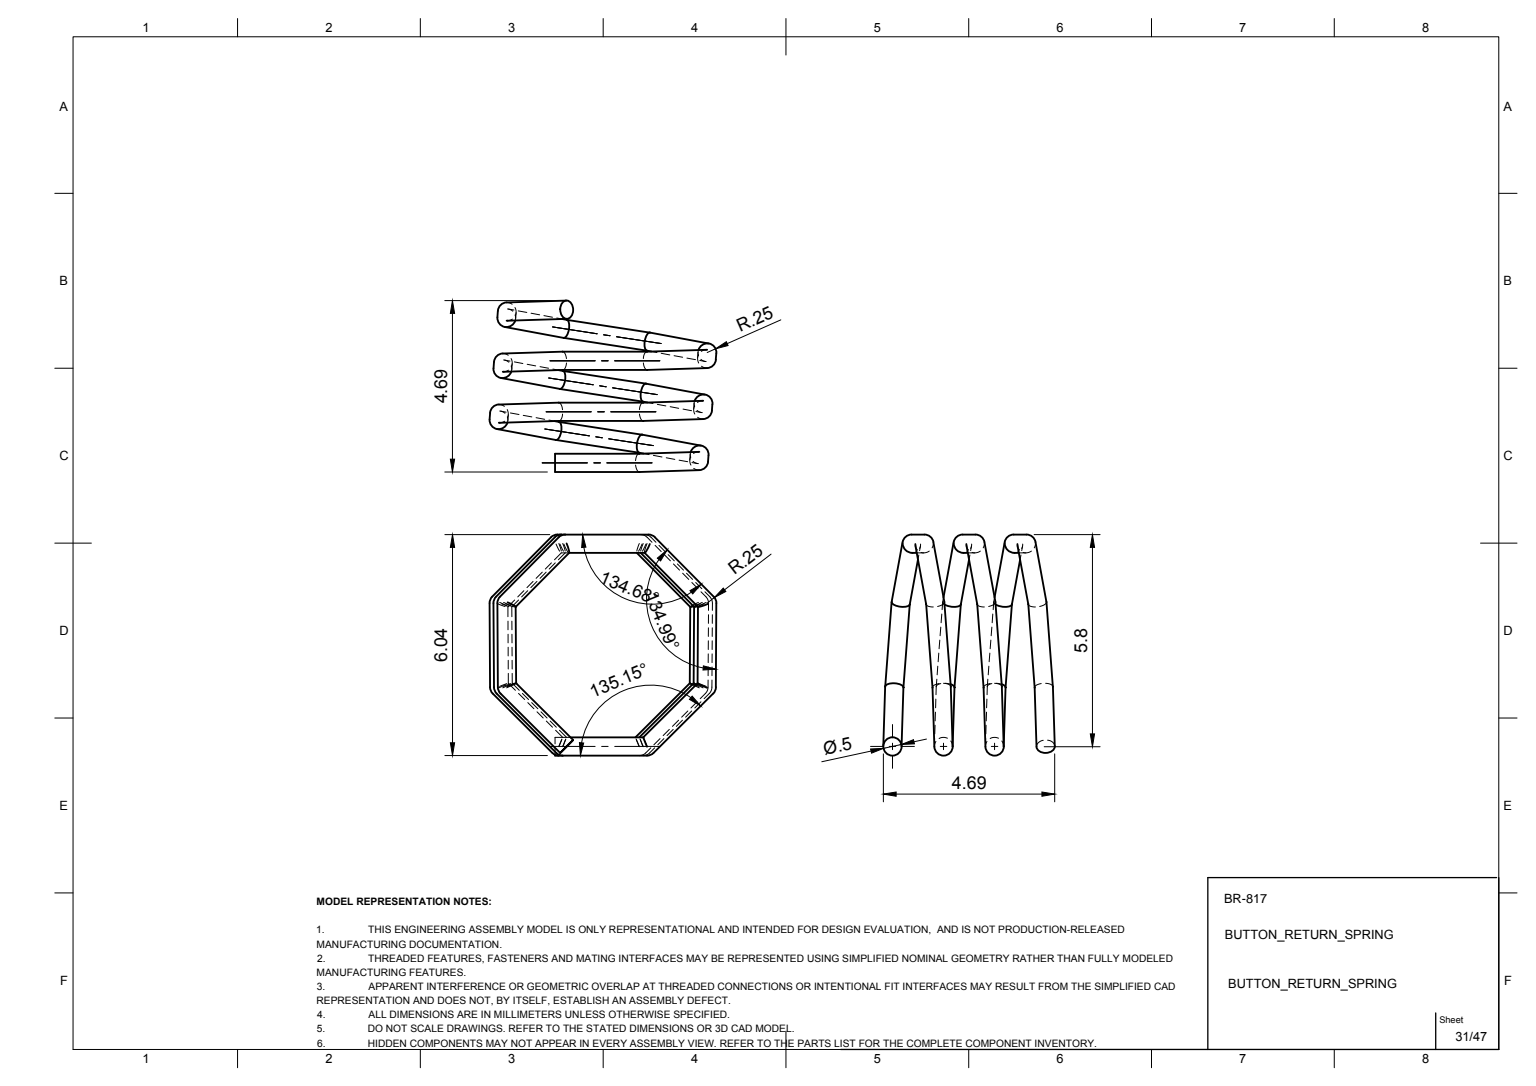
ISO-10303-21;
HEADER;
FILE_DESCRIPTION((''),'2;1');
FILE_NAME('BUTTON_RETURN_SPRING.step','2026-10-01T22:07:29-07:00',(''),(''),'','','');
FILE_SCHEMA (('AUTOMOTIVE_DESIGN { 1 0 10303 214 3 1 1 }'));
ENDSEC;
DATA;
#10=MECHANICAL_DESIGN_GEOMETRIC_PRESENTATION_REPRESENTATION('',(#563),#15484);
#88=ELLIPSE('',#9445,0.0270464082562617,0.025) ;
#89=ELLIPSE('',#9446,0.0270464082562617,0.025) ;
#90=ELLIPSE('',#9447,0.0270464082562617,0.025) ;
#91=ELLIPSE('',#9450,0.0270464082562613,0.025) ;
#92=ELLIPSE('',#9451,0.0270464082562613,0.025) ;
#93=ELLIPSE('',#9453,0.0270464082562612,0.025) ;
#94=ELLIPSE('',#9455,0.0270464082562616,0.025) ;
#95=ELLIPSE('',#9457,0.0270464082562615,0.025) ;
#96=ELLIPSE('',#9459,0.0270464082562615,0.025) ;
#97=ELLIPSE('',#9460,0.0270464082562615,0.025) ;
#98=ELLIPSE('',#9462,0.0270464082562615,0.025) ;
#99=ELLIPSE('',#9463,0.0270464082562615,0.025) ;
#100=ELLIPSE('',#9464,0.0270464082562615,0.025) ;
#101=ELLIPSE('',#9466,0.0270464082562616,0.025) ;
#102=ELLIPSE('',#9467,0.0270464082562616,0.025) ;
#103=ELLIPSE('',#9469,0.0270464082562617,0.025) ;
#104=ELLIPSE('',#9470,0.0270464082562617,0.025) ;
#105=ELLIPSE('',#9471,0.0270464082562617,0.025) ;
#106=ELLIPSE('',#9473,0.0270464082562615,0.025) ;
#107=ELLIPSE('',#9474,0.0270464082562615,0.025) ;
#108=ELLIPSE('',#9476,0.0270464082562614,0.025) ;
#109=ELLIPSE('',#9478,0.0270464082562616,0.025) ;
#110=ELLIPSE('',#9480,0.0270464082562617,0.025) ;
#111=ELLIPSE('',#9482,0.0270464082562615,0.025) ;
#112=ELLIPSE('',#9483,0.0270464082562615,0.025) ;
#113=ELLIPSE('',#9485,0.0270464082562615,0.025) ;
#114=ELLIPSE('',#9486,0.0270464082562615,0.025) ;
#115=ELLIPSE('',#9487,0.0270464082562615,0.025) ;
#116=ELLIPSE('',#9489,0.0270464082562617,0.025) ;
#117=ELLIPSE('',#9490,0.0270464082562617,0.025) ;
#118=ELLIPSE('',#9492,0.0270464082562616,0.025) ;
#119=ELLIPSE('',#9493,0.0270464082562616,0.025) ;
#120=ELLIPSE('',#9494,0.0270464082562616,0.025) ;
#121=ELLIPSE('',#9496,0.0270464082562616,0.025) ;
#122=ELLIPSE('',#9497,0.0270464082562616,0.025) ;
#123=ELLIPSE('',#9499,0.0270464082562614,0.025) ;
#124=ELLIPSE('',#9501,0.0270464082562616,0.025) ;
#125=ELLIPSE('',#9503,0.0270464082562616,0.025) ;
#126=ELLIPSE('',#9505,0.0270464082562616,0.025) ;
#127=ELLIPSE('',#9506,0.0270464082562616,0.025) ;
#128=ELLIPSE('',#9508,0.0270464082562615,0.025) ;
#129=ELLIPSE('',#9509,0.0270464082562615,0.025) ;
#130=ELLIPSE('',#9510,0.0270464082562615,0.025) ;
#237=SPHERICAL_SURFACE('',#9350,0.025) ;
#238=SPHERICAL_SURFACE('',#9353,0.025) ;
#239=SPHERICAL_SURFACE('',#9357,0.025) ;
#240=SPHERICAL_SURFACE('',#9362,0.025) ;
#241=SPHERICAL_SURFACE('',#9367,0.025) ;
#242=SPHERICAL_SURFACE('',#9372,0.025) ;
#243=SPHERICAL_SURFACE('',#9376,0.025) ;
#244=SPHERICAL_SURFACE('',#9379,0.025) ;
#245=SPHERICAL_SURFACE('',#9382,0.025) ;
#246=SPHERICAL_SURFACE('',#9385,0.025) ;
#247=SPHERICAL_SURFACE('',#9389,0.025) ;
#248=SPHERICAL_SURFACE('',#9394,0.025) ;
#249=SPHERICAL_SURFACE('',#9399,0.025) ;
#250=SPHERICAL_SURFACE('',#9404,0.025) ;
#251=SPHERICAL_SURFACE('',#9408,0.025) ;
#252=SPHERICAL_SURFACE('',#9411,0.025) ;
#253=SPHERICAL_SURFACE('',#9414,0.025) ;
#254=SPHERICAL_SURFACE('',#9417,0.025) ;
#255=SPHERICAL_SURFACE('',#9421,0.025) ;
#256=SPHERICAL_SURFACE('',#9426,0.025) ;
#257=SPHERICAL_SURFACE('',#9431,0.025) ;
#258=SPHERICAL_SURFACE('',#9436,0.025) ;
#259=SPHERICAL_SURFACE('',#9440,0.025) ;
#493=SHAPE_REPRESENTATION_RELATIONSHIP('SRR','None',#15643,#528) ;
#528=ADVANCED_BREP_SHAPE_REPRESENTATION('',(#604),#15467) ;
#563=STYLED_ITEM('',(#15832),#604) ;
#604=MANIFOLD_SOLID_BREP('BUTTON_RETURN_SPRING',#8274) ;
#732=CYLINDRICAL_SURFACE('',#9443,0.025) ;
#733=CYLINDRICAL_SURFACE('',#9449,0.025) ;
#734=CYLINDRICAL_SURFACE('',#9452,0.025) ;
#735=CYLINDRICAL_SURFACE('',#9454,0.025) ;
#736=CYLINDRICAL_SURFACE('',#9456,0.025) ;
#737=CYLINDRICAL_SURFACE('',#9458,0.025) ;
#738=CYLINDRICAL_SURFACE('',#9461,0.025) ;
#739=CYLINDRICAL_SURFACE('',#9465,0.025) ;
#740=CYLINDRICAL_SURFACE('',#9468,0.025) ;
#741=CYLINDRICAL_SURFACE('',#9472,0.025) ;
#742=CYLINDRICAL_SURFACE('',#9475,0.025) ;
#743=CYLINDRICAL_SURFACE('',#9477,0.025) ;
#744=CYLINDRICAL_SURFACE('',#9479,0.025) ;
#745=CYLINDRICAL_SURFACE('',#9481,0.025) ;
#746=CYLINDRICAL_SURFACE('',#9484,0.025) ;
#747=CYLINDRICAL_SURFACE('',#9488,0.025) ;
#748=CYLINDRICAL_SURFACE('',#9491,0.025) ;
#749=CYLINDRICAL_SURFACE('',#9495,0.025) ;
#750=CYLINDRICAL_SURFACE('',#9498,0.025) ;
#751=CYLINDRICAL_SURFACE('',#9500,0.025) ;
#752=CYLINDRICAL_SURFACE('',#9502,0.025) ;
#753=CYLINDRICAL_SURFACE('',#9504,0.025) ;
#754=CYLINDRICAL_SURFACE('',#9507,0.025) ;
#755=CYLINDRICAL_SURFACE('',#9511,0.025) ;
#1147=CIRCLE('',#9351,0.025) ;
#1148=CIRCLE('',#9352,0.025) ;
#1149=CIRCLE('',#9354,0.025) ;
#1150=CIRCLE('',#9355,0.025) ;
#1151=CIRCLE('',#9356,0.025) ;
#1152=CIRCLE('',#9358,0.025) ;
#1153=CIRCLE('',#9359,0.025) ;
#1154=CIRCLE('',#9360,0.025) ;
#1155=CIRCLE('',#9361,0.025) ;
#1156=CIRCLE('',#9363,0.025) ;
#1157=CIRCLE('',#9364,0.025) ;
#1158=CIRCLE('',#9365,0.025) ;
#1159=CIRCLE('',#9366,0.025) ;
#1160=CIRCLE('',#9368,0.025) ;
#1161=CIRCLE('',#9369,0.025) ;
#1162=CIRCLE('',#9370,0.025) ;
#1163=CIRCLE('',#9371,0.025) ;
#1164=CIRCLE('',#9373,0.025) ;
#1165=CIRCLE('',#9374,0.025) ;
#1166=CIRCLE('',#9375,0.025) ;
#1167=CIRCLE('',#9377,0.025) ;
#1168=CIRCLE('',#9378,0.025) ;
#1169=CIRCLE('',#9380,0.025) ;
#1170=CIRCLE('',#9381,0.025) ;
#1171=CIRCLE('',#9383,0.025) ;
#1172=CIRCLE('',#9384,0.025) ;
#1173=CIRCLE('',#9386,0.025) ;
#1174=CIRCLE('',#9387,0.025) ;
#1175=CIRCLE('',#9388,0.025) ;
#1176=CIRCLE('',#9390,0.025) ;
#1177=CIRCLE('',#9391,0.025) ;
#1178=CIRCLE('',#9392,0.025) ;
#1179=CIRCLE('',#9393,0.025) ;
#1180=CIRCLE('',#9395,0.025) ;
#1181=CIRCLE('',#9396,0.025) ;
#1182=CIRCLE('',#9397,0.025) ;
#1183=CIRCLE('',#9398,0.025) ;
#1184=CIRCLE('',#9400,0.025) ;
#1185=CIRCLE('',#9401,0.025) ;
#1186=CIRCLE('',#9402,0.025) ;
#1187=CIRCLE('',#9403,0.025) ;
#1188=CIRCLE('',#9405,0.025) ;
#1189=CIRCLE('',#9406,0.025) ;
#1190=CIRCLE('',#9407,0.025) ;
#1191=CIRCLE('',#9409,0.025) ;
#1192=CIRCLE('',#9410,0.025) ;
#1193=CIRCLE('',#9412,0.025) ;
#1194=CIRCLE('',#9413,0.025) ;
#1195=CIRCLE('',#9415,0.025) ;
#1196=CIRCLE('',#9416,0.025) ;
#1197=CIRCLE('',#9418,0.025) ;
#1198=CIRCLE('',#9419,0.025) ;
#1199=CIRCLE('',#9420,0.025) ;
#1200=CIRCLE('',#9422,0.025) ;
#1201=CIRCLE('',#9423,0.025) ;
#1202=CIRCLE('',#9424,0.025) ;
#1203=CIRCLE('',#9425,0.025) ;
#1204=CIRCLE('',#9427,0.025) ;
#1205=CIRCLE('',#9428,0.025) ;
#1206=CIRCLE('',#9429,0.025) ;
#1207=CIRCLE('',#9430,0.025) ;
#1208=CIRCLE('',#9432,0.025) ;
#1209=CIRCLE('',#9433,0.025) ;
#1210=CIRCLE('',#9434,0.025) ;
#1211=CIRCLE('',#9435,0.025) ;
#1212=CIRCLE('',#9437,0.025) ;
#1213=CIRCLE('',#9438,0.025) ;
#1214=CIRCLE('',#9439,0.025) ;
#1215=CIRCLE('',#9441,0.025) ;
#1216=CIRCLE('',#9442,0.025) ;
#1217=CIRCLE('',#9444,0.025) ;
#1218=CIRCLE('',#9512,0.025) ;
#1655=FACE_OUTER_BOUND('',#2220,.T.) ;
#1656=FACE_OUTER_BOUND('',#2221,.T.) ;
#1657=FACE_OUTER_BOUND('',#2222,.T.) ;
#1658=FACE_OUTER_BOUND('',#2223,.T.) ;
#1659=FACE_OUTER_BOUND('',#2224,.T.) ;
#1660=FACE_OUTER_BOUND('',#2225,.T.) ;
#1661=FACE_OUTER_BOUND('',#2226,.T.) ;
#1662=FACE_OUTER_BOUND('',#2227,.T.) ;
#1663=FACE_OUTER_BOUND('',#2228,.T.) ;
#1664=FACE_OUTER_BOUND('',#2229,.T.) ;
#1665=FACE_OUTER_BOUND('',#2230,.T.) ;
#1666=FACE_OUTER_BOUND('',#2231,.T.) ;
#1667=FACE_OUTER_BOUND('',#2232,.T.) ;
#1668=FACE_OUTER_BOUND('',#2233,.T.) ;
#1669=FACE_OUTER_BOUND('',#2234,.T.) ;
#1670=FACE_OUTER_BOUND('',#2235,.T.) ;
#1671=FACE_OUTER_BOUND('',#2236,.T.) ;
#1672=FACE_OUTER_BOUND('',#2237,.T.) ;
#1673=FACE_OUTER_BOUND('',#2238,.T.) ;
#1674=FACE_OUTER_BOUND('',#2239,.T.) ;
#1675=FACE_OUTER_BOUND('',#2240,.T.) ;
#1676=FACE_OUTER_BOUND('',#2241,.T.) ;
#1677=FACE_OUTER_BOUND('',#2242,.T.) ;
#1678=FACE_OUTER_BOUND('',#2243,.T.) ;
#1679=FACE_OUTER_BOUND('',#2244,.T.) ;
#1680=FACE_OUTER_BOUND('',#2245,.T.) ;
#1681=FACE_OUTER_BOUND('',#2246,.T.) ;
#1682=FACE_OUTER_BOUND('',#2247,.T.) ;
#1683=FACE_OUTER_BOUND('',#2248,.T.) ;
#1684=FACE_OUTER_BOUND('',#2249,.T.) ;
#1685=FACE_OUTER_BOUND('',#2250,.T.) ;
#1686=FACE_OUTER_BOUND('',#2251,.T.) ;
#1687=FACE_OUTER_BOUND('',#2252,.T.) ;
#1688=FACE_OUTER_BOUND('',#2253,.T.) ;
#1689=FACE_OUTER_BOUND('',#2254,.T.) ;
#1690=FACE_OUTER_BOUND('',#2255,.T.) ;
#1691=FACE_OUTER_BOUND('',#2256,.T.) ;
#1692=FACE_OUTER_BOUND('',#2257,.T.) ;
#1693=FACE_OUTER_BOUND('',#2258,.T.) ;
#1694=FACE_OUTER_BOUND('',#2259,.T.) ;
#1695=FACE_OUTER_BOUND('',#2260,.T.) ;
#1696=FACE_OUTER_BOUND('',#2261,.T.) ;
#1697=FACE_OUTER_BOUND('',#2262,.T.) ;
#1698=FACE_OUTER_BOUND('',#2263,.T.) ;
#1699=FACE_OUTER_BOUND('',#2264,.T.) ;
#1700=FACE_OUTER_BOUND('',#2265,.T.) ;
#1701=FACE_OUTER_BOUND('',#2266,.T.) ;
#1702=FACE_OUTER_BOUND('',#2267,.T.) ;
#1703=FACE_OUTER_BOUND('',#2268,.T.) ;
#2220=EDGE_LOOP('',(#6565,#6566)) ;
#2221=EDGE_LOOP('',(#6567,#6568,#6569)) ;
#2222=EDGE_LOOP('',(#6570,#6571,#6572,#6573)) ;
#2223=EDGE_LOOP('',(#6574,#6575,#6576,#6577)) ;
#2224=EDGE_LOOP('',(#6578,#6579,#6580,#6581)) ;
#2225=EDGE_LOOP('',(#6582,#6583,#6584)) ;
#2226=EDGE_LOOP('',(#6585,#6586)) ;
#2227=EDGE_LOOP('',(#6587,#6588)) ;
#2228=EDGE_LOOP('',(#6589,#6590)) ;
#2229=EDGE_LOOP('',(#6591,#6592,#6593)) ;
#2230=EDGE_LOOP('',(#6594,#6595,#6596,#6597)) ;
#2231=EDGE_LOOP('',(#6598,#6599,#6600,#6601)) ;
#2232=EDGE_LOOP('',(#6602,#6603,#6604,#6605)) ;
#2233=EDGE_LOOP('',(#6606,#6607,#6608)) ;
#2234=EDGE_LOOP('',(#6609,#6610)) ;
#2235=EDGE_LOOP('',(#6611,#6612)) ;
#2236=EDGE_LOOP('',(#6613,#6614)) ;
#2237=EDGE_LOOP('',(#6615,#6616,#6617)) ;
#2238=EDGE_LOOP('',(#6618,#6619,#6620,#6621)) ;
#2239=EDGE_LOOP('',(#6622,#6623,#6624,#6625)) ;
#2240=EDGE_LOOP('',(#6626,#6627,#6628,#6629)) ;
#2241=EDGE_LOOP('',(#6630,#6631,#6632)) ;
#2242=EDGE_LOOP('',(#6633,#6634)) ;
#2243=EDGE_LOOP('',(#6635,#6636,#6637,#6638,#6639,#6640,#6641)) ;
#2244=EDGE_LOOP('',(#6642)) ;
#2245=EDGE_LOOP('',(#6643,#6644,#6645,#6646,#6647,#6648,#6649,#6650,#6651)) ;
#2246=EDGE_LOOP('',(#6652,#6653,#6654,#6655,#6656,#6657,#6658,#6659,#6660)) ;
#2247=EDGE_LOOP('',(#6661,#6662,#6663,#6664,#6665,#6666,#6667,#6668)) ;
#2248=EDGE_LOOP('',(#6669,#6670,#6671,#6672,#6673,#6674,#6675,#6676)) ;
#2249=EDGE_LOOP('',(#6677,#6678,#6679,#6680,#6681,#6682,#6683,#6684,#6685)) ;
#2250=EDGE_LOOP('',(#6686,#6687,#6688,#6689,#6690,#6691,#6692,#6693,#6694)) ;
#2251=EDGE_LOOP('',(#6695,#6696,#6697,#6698,#6699,#6700,#6701,#6702,#6703)) ;
#2252=EDGE_LOOP('',(#6704,#6705,#6706,#6707,#6708,#6709,#6710,#6711,#6712)) ;
#2253=EDGE_LOOP('',(#6713,#6714,#6715,#6716,#6717,#6718,#6719,#6720,#6721)) ;
#2254=EDGE_LOOP('',(#6722,#6723,#6724,#6725,#6726,#6727,#6728,#6729,#6730)) ;
#2255=EDGE_LOOP('',(#6731,#6732,#6733,#6734,#6735,#6736,#6737,#6738)) ;
#2256=EDGE_LOOP('',(#6739,#6740,#6741,#6742,#6743,#6744,#6745,#6746)) ;
#2257=EDGE_LOOP('',(#6747,#6748,#6749,#6750,#6751,#6752,#6753,#6754,#6755)) ;
#2258=EDGE_LOOP('',(#6756,#6757,#6758,#6759,#6760,#6761,#6762,#6763,#6764)) ;
#2259=EDGE_LOOP('',(#6765,#6766,#6767,#6768,#6769,#6770,#6771,#6772,#6773)) ;
#2260=EDGE_LOOP('',(#6774,#6775,#6776,#6777,#6778,#6779,#6780,#6781,#6782)) ;
#2261=EDGE_LOOP('',(#6783,#6784,#6785,#6786,#6787,#6788,#6789,#6790,#6791)) ;
#2262=EDGE_LOOP('',(#6792,#6793,#6794,#6795,#6796,#6797,#6798,#6799,#6800)) ;
#2263=EDGE_LOOP('',(#6801,#6802,#6803,#6804,#6805,#6806,#6807,#6808)) ;
#2264=EDGE_LOOP('',(#6809,#6810,#6811,#6812,#6813,#6814,#6815,#6816)) ;
#2265=EDGE_LOOP('',(#6817,#6818,#6819,#6820,#6821,#6822,#6823,#6824,#6825)) ;
#2266=EDGE_LOOP('',(#6826,#6827,#6828,#6829,#6830,#6831,#6832,#6833,#6834)) ;
#2267=EDGE_LOOP('',(#6835,#6836,#6837,#6838,#6839,#6840,#6841)) ;
#2268=EDGE_LOOP('',(#6842)) ;
#2747=LINE('',#14502,#3221) ;
#2748=LINE('',#14510,#3222) ;
#2749=LINE('',#14514,#3223) ;
#2750=LINE('',#14517,#3224) ;
#2751=LINE('',#14520,#3225) ;
#2752=LINE('',#14523,#3226) ;
#2753=LINE('',#14529,#3227) ;
#2754=LINE('',#14536,#3228) ;
#2755=LINE('',#14541,#3229) ;
#2756=LINE('',#14548,#3230) ;
#2757=LINE('',#14552,#3231) ;
#2758=LINE('',#14555,#3232) ;
#2759=LINE('',#14558,#3233) ;
#2760=LINE('',#14561,#3234) ;
#2761=LINE('',#14567,#3235) ;
#2762=LINE('',#14574,#3236) ;
#2763=LINE('',#14579,#3237) ;
#2764=LINE('',#14586,#3238) ;
#2765=LINE('',#14590,#3239) ;
#2766=LINE('',#14593,#3240) ;
#2767=LINE('',#14596,#3241) ;
#2768=LINE('',#14599,#3242) ;
#2769=LINE('',#14605,#3243) ;
#2770=LINE('',#14612,#3244) ;
#3221=VECTOR('',#11758,0.025) ;
#3222=VECTOR('',#11769,0.025) ;
#3223=VECTOR('',#11776,0.025) ;
#3224=VECTOR('',#11781,0.025) ;
#3225=VECTOR('',#11786,0.025) ;
#3226=VECTOR('',#11791,0.025) ;
#3227=VECTOR('',#11798,0.025) ;
#3228=VECTOR('',#11807,0.025) ;
#3229=VECTOR('',#11814,0.025) ;
#3230=VECTOR('',#11823,0.025) ;
#3231=VECTOR('',#11830,0.025) ;
#3232=VECTOR('',#11835,0.025) ;
#3233=VECTOR('',#11840,0.025) ;
#3234=VECTOR('',#11845,0.025) ;
#3235=VECTOR('',#11852,0.025) ;
#3236=VECTOR('',#11861,0.025) ;
#3237=VECTOR('',#11868,0.025) ;
#3238=VECTOR('',#11877,0.025) ;
#3239=VECTOR('',#11884,0.025) ;
#3240=VECTOR('',#11889,0.025) ;
#3241=VECTOR('',#11894,0.025) ;
#3242=VECTOR('',#11899,0.025) ;
#3243=VECTOR('',#11906,0.025) ;
#3244=VECTOR('',#11915,0.025) ;
#3819=VERTEX_POINT('',#14336) ;
#3820=VERTEX_POINT('',#14337) ;
#3821=VERTEX_POINT('',#14341) ;
#3822=VERTEX_POINT('',#14342) ;
#3823=VERTEX_POINT('',#14344) ;
#3824=VERTEX_POINT('',#14348) ;
#3825=VERTEX_POINT('',#14349) ;
#3826=VERTEX_POINT('',#14351) ;
#3827=VERTEX_POINT('',#14353) ;
#3828=VERTEX_POINT('',#14357) ;
#3829=VERTEX_POINT('',#14358) ;
#3830=VERTEX_POINT('',#14360) ;
#3831=VERTEX_POINT('',#14362) ;
#3832=VERTEX_POINT('',#14366) ;
#3833=VERTEX_POINT('',#14367) ;
#3834=VERTEX_POINT('',#14369) ;
#3835=VERTEX_POINT('',#14371) ;
#3836=VERTEX_POINT('',#14375) ;
#3837=VERTEX_POINT('',#14376) ;
#3838=VERTEX_POINT('',#14378) ;
#3839=VERTEX_POINT('',#14382) ;
#3840=VERTEX_POINT('',#14383) ;
#3841=VERTEX_POINT('',#14387) ;
#3842=VERTEX_POINT('',#14388) ;
#3843=VERTEX_POINT('',#14392) ;
#3844=VERTEX_POINT('',#14393) ;
#3845=VERTEX_POINT('',#14397) ;
#3846=VERTEX_POINT('',#14398) ;
#3847=VERTEX_POINT('',#14400) ;
#3848=VERTEX_POINT('',#14404) ;
#3849=VERTEX_POINT('',#14405) ;
#3850=VERTEX_POINT('',#14407) ;
#3851=VERTEX_POINT('',#14409) ;
#3852=VERTEX_POINT('',#14413) ;
#3853=VERTEX_POINT('',#14414) ;
#3854=VERTEX_POINT('',#14416) ;
#3855=VERTEX_POINT('',#14418) ;
#3856=VERTEX_POINT('',#14422) ;
#3857=VERTEX_POINT('',#14423) ;
#3858=VERTEX_POINT('',#14425) ;
#3859=VERTEX_POINT('',#14427) ;
#3860=VERTEX_POINT('',#14431) ;
#3861=VERTEX_POINT('',#14432) ;
#3862=VERTEX_POINT('',#14434) ;
#3863=VERTEX_POINT('',#14438) ;
#3864=VERTEX_POINT('',#14439) ;
#3865=VERTEX_POINT('',#14443) ;
#3866=VERTEX_POINT('',#14444) ;
#3867=VERTEX_POINT('',#14448) ;
#3868=VERTEX_POINT('',#14449) ;
#3869=VERTEX_POINT('',#14453) ;
#3870=VERTEX_POINT('',#14454) ;
#3871=VERTEX_POINT('',#14456) ;
#3872=VERTEX_POINT('',#14460) ;
#3873=VERTEX_POINT('',#14461) ;
#3874=VERTEX_POINT('',#14463) ;
#3875=VERTEX_POINT('',#14465) ;
#3876=VERTEX_POINT('',#14469) ;
#3877=VERTEX_POINT('',#14470) ;
#3878=VERTEX_POINT('',#14472) ;
#3879=VERTEX_POINT('',#14474) ;
#3880=VERTEX_POINT('',#14478) ;
#3881=VERTEX_POINT('',#14479) ;
#3882=VERTEX_POINT('',#14481) ;
#3883=VERTEX_POINT('',#14483) ;
#3884=VERTEX_POINT('',#14487) ;
#3885=VERTEX_POINT('',#14488) ;
#3886=VERTEX_POINT('',#14490) ;
#3887=VERTEX_POINT('',#14494) ;
#3888=VERTEX_POINT('',#14495) ;
#3889=VERTEX_POINT('',#14499) ;
#3890=VERTEX_POINT('',#14501) ;
#3891=VERTEX_POINT('',#14503) ;
#3892=VERTEX_POINT('',#14509) ;
#3893=VERTEX_POINT('',#14524) ;
#3894=VERTEX_POINT('',#14528) ;
#3895=VERTEX_POINT('',#14530) ;
#3896=VERTEX_POINT('',#14535) ;
#3897=VERTEX_POINT('',#14540) ;
#3898=VERTEX_POINT('',#14542) ;
#3899=VERTEX_POINT('',#14547) ;
#3900=VERTEX_POINT('',#14562) ;
#3901=VERTEX_POINT('',#14566) ;
#3902=VERTEX_POINT('',#14568) ;
#3903=VERTEX_POINT('',#14573) ;
#3904=VERTEX_POINT('',#14578) ;
#3905=VERTEX_POINT('',#14580) ;
#3906=VERTEX_POINT('',#14585) ;
#3907=VERTEX_POINT('',#14600) ;
#3908=VERTEX_POINT('',#14604) ;
#3909=VERTEX_POINT('',#14606) ;
#3910=VERTEX_POINT('',#14611) ;
#4787=EDGE_CURVE('',#3819,#3820,#1147,.T.) ;
#4788=EDGE_CURVE('',#3820,#3819,#1148,.T.) ;
#4789=EDGE_CURVE('',#3821,#3822,#1149,.T.) ;
#4790=EDGE_CURVE('',#3822,#3823,#1150,.T.) ;
#4791=EDGE_CURVE('',#3823,#3821,#1151,.T.) ;
#4792=EDGE_CURVE('',#3824,#3825,#1152,.T.) ;
#4793=EDGE_CURVE('',#3825,#3826,#1153,.T.) ;
#4794=EDGE_CURVE('',#3826,#3827,#1154,.T.) ;
#4795=EDGE_CURVE('',#3827,#3824,#1155,.T.) ;
#4796=EDGE_CURVE('',#3828,#3829,#1156,.T.) ;
#4797=EDGE_CURVE('',#3829,#3830,#1157,.T.) ;
#4798=EDGE_CURVE('',#3830,#3831,#1158,.T.) ;
#4799=EDGE_CURVE('',#3831,#3828,#1159,.T.) ;
#4800=EDGE_CURVE('',#3832,#3833,#1160,.T.) ;
#4801=EDGE_CURVE('',#3833,#3834,#1161,.T.) ;
#4802=EDGE_CURVE('',#3834,#3835,#1162,.T.) ;
#4803=EDGE_CURVE('',#3835,#3832,#1163,.T.) ;
#4804=EDGE_CURVE('',#3836,#3837,#1164,.T.) ;
#4805=EDGE_CURVE('',#3837,#3838,#1165,.T.) ;
#4806=EDGE_CURVE('',#3838,#3836,#1166,.T.) ;
#4807=EDGE_CURVE('',#3839,#3840,#1167,.T.) ;
#4808=EDGE_CURVE('',#3840,#3839,#1168,.T.) ;
#4809=EDGE_CURVE('',#3841,#3842,#1169,.T.) ;
#4810=EDGE_CURVE('',#3842,#3841,#1170,.T.) ;
#4811=EDGE_CURVE('',#3843,#3844,#1171,.T.) ;
#4812=EDGE_CURVE('',#3844,#3843,#1172,.T.) ;
#4813=EDGE_CURVE('',#3845,#3846,#1173,.T.) ;
#4814=EDGE_CURVE('',#3846,#3847,#1174,.T.) ;
#4815=EDGE_CURVE('',#3847,#3845,#1175,.T.) ;
#4816=EDGE_CURVE('',#3848,#3849,#1176,.T.) ;
#4817=EDGE_CURVE('',#3849,#3850,#1177,.T.) ;
#4818=EDGE_CURVE('',#3850,#3851,#1178,.T.) ;
#4819=EDGE_CURVE('',#3851,#3848,#1179,.T.) ;
#4820=EDGE_CURVE('',#3852,#3853,#1180,.T.) ;
#4821=EDGE_CURVE('',#3853,#3854,#1181,.T.) ;
#4822=EDGE_CURVE('',#3854,#3855,#1182,.T.) ;
#4823=EDGE_CURVE('',#3855,#3852,#1183,.T.) ;
#4824=EDGE_CURVE('',#3856,#3857,#1184,.T.) ;
#4825=EDGE_CURVE('',#3857,#3858,#1185,.T.) ;
#4826=EDGE_CURVE('',#3858,#3859,#1186,.T.) ;
#4827=EDGE_CURVE('',#3859,#3856,#1187,.T.) ;
#4828=EDGE_CURVE('',#3860,#3861,#1188,.T.) ;
#4829=EDGE_CURVE('',#3861,#3862,#1189,.T.) ;
#4830=EDGE_CURVE('',#3862,#3860,#1190,.T.) ;
#4831=EDGE_CURVE('',#3863,#3864,#1191,.T.) ;
#4832=EDGE_CURVE('',#3864,#3863,#1192,.T.) ;
#4833=EDGE_CURVE('',#3865,#3866,#1193,.T.) ;
#4834=EDGE_CURVE('',#3866,#3865,#1194,.T.) ;
#4835=EDGE_CURVE('',#3867,#3868,#1195,.T.) ;
#4836=EDGE_CURVE('',#3868,#3867,#1196,.T.) ;
#4837=EDGE_CURVE('',#3869,#3870,#1197,.T.) ;
#4838=EDGE_CURVE('',#3870,#3871,#1198,.T.) ;
#4839=EDGE_CURVE('',#3871,#3869,#1199,.T.) ;
#4840=EDGE_CURVE('',#3872,#3873,#1200,.T.) ;
#4841=EDGE_CURVE('',#3873,#3874,#1201,.T.) ;
#4842=EDGE_CURVE('',#3874,#3875,#1202,.T.) ;
#4843=EDGE_CURVE('',#3875,#3872,#1203,.T.) ;
#4844=EDGE_CURVE('',#3876,#3877,#1204,.T.) ;
#4845=EDGE_CURVE('',#3877,#3878,#1205,.T.) ;
#4846=EDGE_CURVE('',#3878,#3879,#1206,.T.) ;
#4847=EDGE_CURVE('',#3879,#3876,#1207,.T.) ;
#4848=EDGE_CURVE('',#3880,#3881,#1208,.T.) ;
#4849=EDGE_CURVE('',#3881,#3882,#1209,.T.) ;
#4850=EDGE_CURVE('',#3882,#3883,#1210,.T.) ;
#4851=EDGE_CURVE('',#3883,#3880,#1211,.T.) ;
#4852=EDGE_CURVE('',#3884,#3885,#1212,.T.) ;
#4853=EDGE_CURVE('',#3885,#3886,#1213,.T.) ;
#4854=EDGE_CURVE('',#3886,#3884,#1214,.T.) ;
#4855=EDGE_CURVE('',#3887,#3888,#1215,.T.) ;
#4856=EDGE_CURVE('',#3888,#3887,#1216,.T.) ;
#4857=EDGE_CURVE('',#3889,#3889,#1217,.T.) ;
#4858=EDGE_CURVE('',#3889,#3890,#2747,.T.) ;
#4859=EDGE_CURVE('',#3891,#3890,#88,.T.) ;
#4860=EDGE_CURVE('',#3820,#3891,#89,.T.) ;
#4861=EDGE_CURVE('',#3890,#3819,#90,.T.) ;
#4862=EDGE_CURVE('',#3891,#3892,#2748,.T.) ;
#4863=EDGE_CURVE('',#3822,#3892,#91,.T.) ;
#4864=EDGE_CURVE('',#3892,#3821,#92,.T.) ;
#4865=EDGE_CURVE('',#3823,#3825,#2749,.T.) ;
#4866=EDGE_CURVE('',#3826,#3824,#93,.T.) ;
#4867=EDGE_CURVE('',#3827,#3829,#2750,.T.) ;
#4868=EDGE_CURVE('',#3830,#3828,#94,.T.) ;
#4869=EDGE_CURVE('',#3831,#3833,#2751,.T.) ;
#4870=EDGE_CURVE('',#3834,#3832,#95,.T.) ;
#4871=EDGE_CURVE('',#3835,#3837,#2752,.T.) ;
#4872=EDGE_CURVE('',#3893,#3836,#96,.T.) ;
#4873=EDGE_CURVE('',#3838,#3893,#97,.T.) ;
#4874=EDGE_CURVE('',#3893,#3894,#2753,.T.) ;
#4875=EDGE_CURVE('',#3895,#3894,#98,.T.) ;
#4876=EDGE_CURVE('',#3840,#3895,#99,.T.) ;
#4877=EDGE_CURVE('',#3894,#3839,#100,.T.) ;
#4878=EDGE_CURVE('',#3895,#3896,#2754,.T.) ;
#4879=EDGE_CURVE('',#3842,#3896,#101,.T.) ;
#4880=EDGE_CURVE('',#3896,#3841,#102,.T.) ;
#4881=EDGE_CURVE('',#3896,#3897,#2755,.T.) ;
#4882=EDGE_CURVE('',#3898,#3897,#103,.T.) ;
#4883=EDGE_CURVE('',#3844,#3898,#104,.T.) ;
#4884=EDGE_CURVE('',#3897,#3843,#105,.T.) ;
#4885=EDGE_CURVE('',#3898,#3899,#2756,.T.) ;
#4886=EDGE_CURVE('',#3846,#3899,#106,.T.) ;
#4887=EDGE_CURVE('',#3899,#3845,#107,.T.) ;
#4888=EDGE_CURVE('',#3847,#3849,#2757,.T.) ;
#4889=EDGE_CURVE('',#3850,#3848,#108,.T.) ;
#4890=EDGE_CURVE('',#3851,#3853,#2758,.T.) ;
#4891=EDGE_CURVE('',#3854,#3852,#109,.T.) ;
#4892=EDGE_CURVE('',#3855,#3857,#2759,.T.) ;
#4893=EDGE_CURVE('',#3858,#3856,#110,.T.) ;
#4894=EDGE_CURVE('',#3859,#3861,#2760,.T.) ;
#4895=EDGE_CURVE('',#3900,#3860,#111,.T.) ;
#4896=EDGE_CURVE('',#3862,#3900,#112,.T.) ;
#4897=EDGE_CURVE('',#3900,#3901,#2761,.T.) ;
#4898=EDGE_CURVE('',#3902,#3901,#113,.T.) ;
#4899=EDGE_CURVE('',#3864,#3902,#114,.T.) ;
#4900=EDGE_CURVE('',#3901,#3863,#115,.T.) ;
#4901=EDGE_CURVE('',#3902,#3903,#2762,.T.) ;
#4902=EDGE_CURVE('',#3866,#3903,#116,.T.) ;
#4903=EDGE_CURVE('',#3903,#3865,#117,.T.) ;
#4904=EDGE_CURVE('',#3903,#3904,#2763,.T.) ;
#4905=EDGE_CURVE('',#3905,#3904,#118,.T.) ;
#4906=EDGE_CURVE('',#3868,#3905,#119,.T.) ;
#4907=EDGE_CURVE('',#3904,#3867,#120,.T.) ;
#4908=EDGE_CURVE('',#3905,#3906,#2764,.T.) ;
#4909=EDGE_CURVE('',#3870,#3906,#121,.T.) ;
#4910=EDGE_CURVE('',#3906,#3869,#122,.T.) ;
#4911=EDGE_CURVE('',#3871,#3873,#2765,.T.) ;
#4912=EDGE_CURVE('',#3874,#3872,#123,.T.) ;
#4913=EDGE_CURVE('',#3875,#3877,#2766,.T.) ;
#4914=EDGE_CURVE('',#3878,#3876,#124,.T.) ;
#4915=EDGE_CURVE('',#3879,#3881,#2767,.T.) ;
#4916=EDGE_CURVE('',#3882,#3880,#125,.T.) ;
#4917=EDGE_CURVE('',#3883,#3885,#2768,.T.) ;
#4918=EDGE_CURVE('',#3907,#3884,#126,.T.) ;
#4919=EDGE_CURVE('',#3886,#3907,#127,.T.) ;
#4920=EDGE_CURVE('',#3907,#3908,#2769,.T.) ;
#4921=EDGE_CURVE('',#3909,#3908,#128,.T.) ;
#4922=EDGE_CURVE('',#3888,#3909,#129,.T.) ;
#4923=EDGE_CURVE('',#3908,#3887,#130,.T.) ;
#4924=EDGE_CURVE('',#3909,#3910,#2770,.T.) ;
#4925=EDGE_CURVE('',#3910,#3910,#1218,.T.) ;
#6565=ORIENTED_EDGE('',*,*,#4787,.T.) ;
#6566=ORIENTED_EDGE('',*,*,#4788,.T.) ;
#6567=ORIENTED_EDGE('',*,*,#4789,.T.) ;
#6568=ORIENTED_EDGE('',*,*,#4790,.T.) ;
#6569=ORIENTED_EDGE('',*,*,#4791,.T.) ;
#6570=ORIENTED_EDGE('',*,*,#4792,.T.) ;
#6571=ORIENTED_EDGE('',*,*,#4793,.T.) ;
#6572=ORIENTED_EDGE('',*,*,#4794,.T.) ;
#6573=ORIENTED_EDGE('',*,*,#4795,.T.) ;
#6574=ORIENTED_EDGE('',*,*,#4796,.T.) ;
#6575=ORIENTED_EDGE('',*,*,#4797,.T.) ;
#6576=ORIENTED_EDGE('',*,*,#4798,.T.) ;
#6577=ORIENTED_EDGE('',*,*,#4799,.T.) ;
#6578=ORIENTED_EDGE('',*,*,#4800,.T.) ;
#6579=ORIENTED_EDGE('',*,*,#4801,.T.) ;
#6580=ORIENTED_EDGE('',*,*,#4802,.T.) ;
#6581=ORIENTED_EDGE('',*,*,#4803,.T.) ;
#6582=ORIENTED_EDGE('',*,*,#4804,.T.) ;
#6583=ORIENTED_EDGE('',*,*,#4805,.T.) ;
#6584=ORIENTED_EDGE('',*,*,#4806,.T.) ;
#6585=ORIENTED_EDGE('',*,*,#4807,.T.) ;
#6586=ORIENTED_EDGE('',*,*,#4808,.T.) ;
#6587=ORIENTED_EDGE('',*,*,#4809,.T.) ;
#6588=ORIENTED_EDGE('',*,*,#4810,.T.) ;
#6589=ORIENTED_EDGE('',*,*,#4811,.T.) ;
#6590=ORIENTED_EDGE('',*,*,#4812,.T.) ;
#6591=ORIENTED_EDGE('',*,*,#4813,.T.) ;
#6592=ORIENTED_EDGE('',*,*,#4814,.T.) ;
#6593=ORIENTED_EDGE('',*,*,#4815,.T.) ;
#6594=ORIENTED_EDGE('',*,*,#4816,.T.) ;
#6595=ORIENTED_EDGE('',*,*,#4817,.T.) ;
#6596=ORIENTED_EDGE('',*,*,#4818,.T.) ;
#6597=ORIENTED_EDGE('',*,*,#4819,.T.) ;
#6598=ORIENTED_EDGE('',*,*,#4820,.T.) ;
#6599=ORIENTED_EDGE('',*,*,#4821,.T.) ;
#6600=ORIENTED_EDGE('',*,*,#4822,.T.) ;
#6601=ORIENTED_EDGE('',*,*,#4823,.T.) ;
#6602=ORIENTED_EDGE('',*,*,#4824,.T.) ;
#6603=ORIENTED_EDGE('',*,*,#4825,.T.) ;
#6604=ORIENTED_EDGE('',*,*,#4826,.T.) ;
#6605=ORIENTED_EDGE('',*,*,#4827,.T.) ;
#6606=ORIENTED_EDGE('',*,*,#4828,.T.) ;
#6607=ORIENTED_EDGE('',*,*,#4829,.T.) ;
#6608=ORIENTED_EDGE('',*,*,#4830,.T.) ;
#6609=ORIENTED_EDGE('',*,*,#4831,.T.) ;
#6610=ORIENTED_EDGE('',*,*,#4832,.T.) ;
#6611=ORIENTED_EDGE('',*,*,#4833,.T.) ;
#6612=ORIENTED_EDGE('',*,*,#4834,.T.) ;
#6613=ORIENTED_EDGE('',*,*,#4835,.T.) ;
#6614=ORIENTED_EDGE('',*,*,#4836,.T.) ;
#6615=ORIENTED_EDGE('',*,*,#4837,.T.) ;
#6616=ORIENTED_EDGE('',*,*,#4838,.T.) ;
#6617=ORIENTED_EDGE('',*,*,#4839,.T.) ;
#6618=ORIENTED_EDGE('',*,*,#4840,.T.) ;
#6619=ORIENTED_EDGE('',*,*,#4841,.T.) ;
#6620=ORIENTED_EDGE('',*,*,#4842,.T.) ;
#6621=ORIENTED_EDGE('',*,*,#4843,.T.) ;
#6622=ORIENTED_EDGE('',*,*,#4844,.T.) ;
#6623=ORIENTED_EDGE('',*,*,#4845,.T.) ;
#6624=ORIENTED_EDGE('',*,*,#4846,.T.) ;
#6625=ORIENTED_EDGE('',*,*,#4847,.T.) ;
#6626=ORIENTED_EDGE('',*,*,#4848,.T.) ;
#6627=ORIENTED_EDGE('',*,*,#4849,.T.) ;
#6628=ORIENTED_EDGE('',*,*,#4850,.T.) ;
#6629=ORIENTED_EDGE('',*,*,#4851,.T.) ;
#6630=ORIENTED_EDGE('',*,*,#4852,.T.) ;
#6631=ORIENTED_EDGE('',*,*,#4853,.T.) ;
#6632=ORIENTED_EDGE('',*,*,#4854,.T.) ;
#6633=ORIENTED_EDGE('',*,*,#4855,.T.) ;
#6634=ORIENTED_EDGE('',*,*,#4856,.T.) ;
#6635=ORIENTED_EDGE('',*,*,#4857,.F.) ;
#6636=ORIENTED_EDGE('',*,*,#4858,.T.) ;
#6637=ORIENTED_EDGE('',*,*,#4859,.F.) ;
#6638=ORIENTED_EDGE('',*,*,#4860,.F.) ;
#6639=ORIENTED_EDGE('',*,*,#4787,.F.) ;
#6640=ORIENTED_EDGE('',*,*,#4861,.F.) ;
#6641=ORIENTED_EDGE('',*,*,#4858,.F.) ;
#6642=ORIENTED_EDGE('',*,*,#4857,.T.) ;
#6643=ORIENTED_EDGE('',*,*,#4860,.T.) ;
#6644=ORIENTED_EDGE('',*,*,#4862,.T.) ;
#6645=ORIENTED_EDGE('',*,*,#4863,.F.) ;
#6646=ORIENTED_EDGE('',*,*,#4789,.F.) ;
#6647=ORIENTED_EDGE('',*,*,#4864,.F.) ;
#6648=ORIENTED_EDGE('',*,*,#4862,.F.) ;
#6649=ORIENTED_EDGE('',*,*,#4859,.T.) ;
#6650=ORIENTED_EDGE('',*,*,#4861,.T.) ;
#6651=ORIENTED_EDGE('',*,*,#4788,.F.) ;
#6652=ORIENTED_EDGE('',*,*,#4863,.T.) ;
#6653=ORIENTED_EDGE('',*,*,#4864,.T.) ;
#6654=ORIENTED_EDGE('',*,*,#4791,.F.) ;
#6655=ORIENTED_EDGE('',*,*,#4865,.T.) ;
#6656=ORIENTED_EDGE('',*,*,#4792,.F.) ;
#6657=ORIENTED_EDGE('',*,*,#4866,.F.) ;
#6658=ORIENTED_EDGE('',*,*,#4793,.F.) ;
#6659=ORIENTED_EDGE('',*,*,#4865,.F.) ;
#6660=ORIENTED_EDGE('',*,*,#4790,.F.) ;
#6661=ORIENTED_EDGE('',*,*,#4866,.T.) ;
#6662=ORIENTED_EDGE('',*,*,#4795,.F.) ;
#6663=ORIENTED_EDGE('',*,*,#4867,.T.) ;
#6664=ORIENTED_EDGE('',*,*,#4796,.F.) ;
#6665=ORIENTED_EDGE('',*,*,#4868,.F.) ;
#6666=ORIENTED_EDGE('',*,*,#4797,.F.) ;
#6667=ORIENTED_EDGE('',*,*,#4867,.F.) ;
#6668=ORIENTED_EDGE('',*,*,#4794,.F.) ;
#6669=ORIENTED_EDGE('',*,*,#4868,.T.) ;
#6670=ORIENTED_EDGE('',*,*,#4799,.F.) ;
#6671=ORIENTED_EDGE('',*,*,#4869,.T.) ;
#6672=ORIENTED_EDGE('',*,*,#4800,.F.) ;
#6673=ORIENTED_EDGE('',*,*,#4870,.F.) ;
#6674=ORIENTED_EDGE('',*,*,#4801,.F.) ;
#6675=ORIENTED_EDGE('',*,*,#4869,.F.) ;
#6676=ORIENTED_EDGE('',*,*,#4798,.F.) ;
#6677=ORIENTED_EDGE('',*,*,#4870,.T.) ;
#6678=ORIENTED_EDGE('',*,*,#4803,.F.) ;
#6679=ORIENTED_EDGE('',*,*,#4871,.T.) ;
#6680=ORIENTED_EDGE('',*,*,#4804,.F.) ;
#6681=ORIENTED_EDGE('',*,*,#4872,.F.) ;
#6682=ORIENTED_EDGE('',*,*,#4873,.F.) ;
#6683=ORIENTED_EDGE('',*,*,#4805,.F.) ;
#6684=ORIENTED_EDGE('',*,*,#4871,.F.) ;
#6685=ORIENTED_EDGE('',*,*,#4802,.F.) ;
#6686=ORIENTED_EDGE('',*,*,#4873,.T.) ;
#6687=ORIENTED_EDGE('',*,*,#4874,.T.) ;
#6688=ORIENTED_EDGE('',*,*,#4875,.F.) ;
#6689=ORIENTED_EDGE('',*,*,#4876,.F.) ;
#6690=ORIENTED_EDGE('',*,*,#4807,.F.) ;
#6691=ORIENTED_EDGE('',*,*,#4877,.F.) ;
#6692=ORIENTED_EDGE('',*,*,#4874,.F.) ;
#6693=ORIENTED_EDGE('',*,*,#4872,.T.) ;
#6694=ORIENTED_EDGE('',*,*,#4806,.F.) ;
#6695=ORIENTED_EDGE('',*,*,#4876,.T.) ;
#6696=ORIENTED_EDGE('',*,*,#4878,.T.) ;
#6697=ORIENTED_EDGE('',*,*,#4879,.F.) ;
#6698=ORIENTED_EDGE('',*,*,#4809,.F.) ;
#6699=ORIENTED_EDGE('',*,*,#4880,.F.) ;
#6700=ORIENTED_EDGE('',*,*,#4878,.F.) ;
#6701=ORIENTED_EDGE('',*,*,#4875,.T.) ;
#6702=ORIENTED_EDGE('',*,*,#4877,.T.) ;
#6703=ORIENTED_EDGE('',*,*,#4808,.F.) ;
#6704=ORIENTED_EDGE('',*,*,#4879,.T.) ;
#6705=ORIENTED_EDGE('',*,*,#4881,.T.) ;
#6706=ORIENTED_EDGE('',*,*,#4882,.F.) ;
#6707=ORIENTED_EDGE('',*,*,#4883,.F.) ;
#6708=ORIENTED_EDGE('',*,*,#4811,.F.) ;
#6709=ORIENTED_EDGE('',*,*,#4884,.F.) ;
#6710=ORIENTED_EDGE('',*,*,#4881,.F.) ;
#6711=ORIENTED_EDGE('',*,*,#4880,.T.) ;
#6712=ORIENTED_EDGE('',*,*,#4810,.F.) ;
#6713=ORIENTED_EDGE('',*,*,#4883,.T.) ;
#6714=ORIENTED_EDGE('',*,*,#4885,.T.) ;
#6715=ORIENTED_EDGE('',*,*,#4886,.F.) ;
#6716=ORIENTED_EDGE('',*,*,#4813,.F.) ;
#6717=ORIENTED_EDGE('',*,*,#4887,.F.) ;
#6718=ORIENTED_EDGE('',*,*,#4885,.F.) ;
#6719=ORIENTED_EDGE('',*,*,#4882,.T.) ;
#6720=ORIENTED_EDGE('',*,*,#4884,.T.) ;
#6721=ORIENTED_EDGE('',*,*,#4812,.F.) ;
#6722=ORIENTED_EDGE('',*,*,#4886,.T.) ;
#6723=ORIENTED_EDGE('',*,*,#4887,.T.) ;
#6724=ORIENTED_EDGE('',*,*,#4815,.F.) ;
#6725=ORIENTED_EDGE('',*,*,#4888,.T.) ;
#6726=ORIENTED_EDGE('',*,*,#4816,.F.) ;
#6727=ORIENTED_EDGE('',*,*,#4889,.F.) ;
#6728=ORIENTED_EDGE('',*,*,#4817,.F.) ;
#6729=ORIENTED_EDGE('',*,*,#4888,.F.) ;
#6730=ORIENTED_EDGE('',*,*,#4814,.F.) ;
#6731=ORIENTED_EDGE('',*,*,#4889,.T.) ;
#6732=ORIENTED_EDGE('',*,*,#4819,.F.) ;
#6733=ORIENTED_EDGE('',*,*,#4890,.T.) ;
#6734=ORIENTED_EDGE('',*,*,#4820,.F.) ;
#6735=ORIENTED_EDGE('',*,*,#4891,.F.) ;
#6736=ORIENTED_EDGE('',*,*,#4821,.F.) ;
#6737=ORIENTED_EDGE('',*,*,#4890,.F.) ;
#6738=ORIENTED_EDGE('',*,*,#4818,.F.) ;
#6739=ORIENTED_EDGE('',*,*,#4891,.T.) ;
#6740=ORIENTED_EDGE('',*,*,#4823,.F.) ;
#6741=ORIENTED_EDGE('',*,*,#4892,.T.) ;
#6742=ORIENTED_EDGE('',*,*,#4824,.F.) ;
#6743=ORIENTED_EDGE('',*,*,#4893,.F.) ;
#6744=ORIENTED_EDGE('',*,*,#4825,.F.) ;
#6745=ORIENTED_EDGE('',*,*,#4892,.F.) ;
#6746=ORIENTED_EDGE('',*,*,#4822,.F.) ;
#6747=ORIENTED_EDGE('',*,*,#4893,.T.) ;
#6748=ORIENTED_EDGE('',*,*,#4827,.F.) ;
#6749=ORIENTED_EDGE('',*,*,#4894,.T.) ;
#6750=ORIENTED_EDGE('',*,*,#4828,.F.) ;
#6751=ORIENTED_EDGE('',*,*,#4895,.F.) ;
#6752=ORIENTED_EDGE('',*,*,#4896,.F.) ;
#6753=ORIENTED_EDGE('',*,*,#4829,.F.) ;
#6754=ORIENTED_EDGE('',*,*,#4894,.F.) ;
#6755=ORIENTED_EDGE('',*,*,#4826,.F.) ;
#6756=ORIENTED_EDGE('',*,*,#4896,.T.) ;
#6757=ORIENTED_EDGE('',*,*,#4897,.T.) ;
#6758=ORIENTED_EDGE('',*,*,#4898,.F.) ;
#6759=ORIENTED_EDGE('',*,*,#4899,.F.) ;
#6760=ORIENTED_EDGE('',*,*,#4831,.F.) ;
#6761=ORIENTED_EDGE('',*,*,#4900,.F.) ;
#6762=ORIENTED_EDGE('',*,*,#4897,.F.) ;
#6763=ORIENTED_EDGE('',*,*,#4895,.T.) ;
#6764=ORIENTED_EDGE('',*,*,#4830,.F.) ;
#6765=ORIENTED_EDGE('',*,*,#4899,.T.) ;
#6766=ORIENTED_EDGE('',*,*,#4901,.T.) ;
#6767=ORIENTED_EDGE('',*,*,#4902,.F.) ;
#6768=ORIENTED_EDGE('',*,*,#4833,.F.) ;
#6769=ORIENTED_EDGE('',*,*,#4903,.F.) ;
#6770=ORIENTED_EDGE('',*,*,#4901,.F.) ;
#6771=ORIENTED_EDGE('',*,*,#4898,.T.) ;
#6772=ORIENTED_EDGE('',*,*,#4900,.T.) ;
#6773=ORIENTED_EDGE('',*,*,#4832,.F.) ;
#6774=ORIENTED_EDGE('',*,*,#4902,.T.) ;
#6775=ORIENTED_EDGE('',*,*,#4904,.T.) ;
#6776=ORIENTED_EDGE('',*,*,#4905,.F.) ;
#6777=ORIENTED_EDGE('',*,*,#4906,.F.) ;
#6778=ORIENTED_EDGE('',*,*,#4835,.F.) ;
#6779=ORIENTED_EDGE('',*,*,#4907,.F.) ;
#6780=ORIENTED_EDGE('',*,*,#4904,.F.) ;
#6781=ORIENTED_EDGE('',*,*,#4903,.T.) ;
#6782=ORIENTED_EDGE('',*,*,#4834,.F.) ;
#6783=ORIENTED_EDGE('',*,*,#4906,.T.) ;
#6784=ORIENTED_EDGE('',*,*,#4908,.T.) ;
#6785=ORIENTED_EDGE('',*,*,#4909,.F.) ;
#6786=ORIENTED_EDGE('',*,*,#4837,.F.) ;
#6787=ORIENTED_EDGE('',*,*,#4910,.F.) ;
#6788=ORIENTED_EDGE('',*,*,#4908,.F.) ;
#6789=ORIENTED_EDGE('',*,*,#4905,.T.) ;
#6790=ORIENTED_EDGE('',*,*,#4907,.T.) ;
#6791=ORIENTED_EDGE('',*,*,#4836,.F.) ;
#6792=ORIENTED_EDGE('',*,*,#4909,.T.) ;
#6793=ORIENTED_EDGE('',*,*,#4910,.T.) ;
#6794=ORIENTED_EDGE('',*,*,#4839,.F.) ;
#6795=ORIENTED_EDGE('',*,*,#4911,.T.) ;
#6796=ORIENTED_EDGE('',*,*,#4840,.F.) ;
#6797=ORIENTED_EDGE('',*,*,#4912,.F.) ;
#6798=ORIENTED_EDGE('',*,*,#4841,.F.) ;
#6799=ORIENTED_EDGE('',*,*,#4911,.F.) ;
#6800=ORIENTED_EDGE('',*,*,#4838,.F.) ;
#6801=ORIENTED_EDGE('',*,*,#4912,.T.) ;
#6802=ORIENTED_EDGE('',*,*,#4843,.F.) ;
#6803=ORIENTED_EDGE('',*,*,#4913,.T.) ;
#6804=ORIENTED_EDGE('',*,*,#4844,.F.) ;
#6805=ORIENTED_EDGE('',*,*,#4914,.F.) ;
#6806=ORIENTED_EDGE('',*,*,#4845,.F.) ;
#6807=ORIENTED_EDGE('',*,*,#4913,.F.) ;
#6808=ORIENTED_EDGE('',*,*,#4842,.F.) ;
#6809=ORIENTED_EDGE('',*,*,#4914,.T.) ;
#6810=ORIENTED_EDGE('',*,*,#4847,.F.) ;
#6811=ORIENTED_EDGE('',*,*,#4915,.T.) ;
#6812=ORIENTED_EDGE('',*,*,#4848,.F.) ;
#6813=ORIENTED_EDGE('',*,*,#4916,.F.) ;
#6814=ORIENTED_EDGE('',*,*,#4849,.F.) ;
#6815=ORIENTED_EDGE('',*,*,#4915,.F.) ;
#6816=ORIENTED_EDGE('',*,*,#4846,.F.) ;
#6817=ORIENTED_EDGE('',*,*,#4916,.T.) ;
#6818=ORIENTED_EDGE('',*,*,#4851,.F.) ;
#6819=ORIENTED_EDGE('',*,*,#4917,.T.) ;
#6820=ORIENTED_EDGE('',*,*,#4852,.F.) ;
#6821=ORIENTED_EDGE('',*,*,#4918,.F.) ;
#6822=ORIENTED_EDGE('',*,*,#4919,.F.) ;
#6823=ORIENTED_EDGE('',*,*,#4853,.F.) ;
#6824=ORIENTED_EDGE('',*,*,#4917,.F.) ;
#6825=ORIENTED_EDGE('',*,*,#4850,.F.) ;
#6826=ORIENTED_EDGE('',*,*,#4919,.T.) ;
#6827=ORIENTED_EDGE('',*,*,#4920,.T.) ;
#6828=ORIENTED_EDGE('',*,*,#4921,.F.) ;
#6829=ORIENTED_EDGE('',*,*,#4922,.F.) ;
#6830=ORIENTED_EDGE('',*,*,#4855,.F.) ;
#6831=ORIENTED_EDGE('',*,*,#4923,.F.) ;
#6832=ORIENTED_EDGE('',*,*,#4920,.F.) ;
#6833=ORIENTED_EDGE('',*,*,#4918,.T.) ;
#6834=ORIENTED_EDGE('',*,*,#4854,.F.) ;
#6835=ORIENTED_EDGE('',*,*,#4922,.T.) ;
#6836=ORIENTED_EDGE('',*,*,#4924,.T.) ;
#6837=ORIENTED_EDGE('',*,*,#4925,.F.) ;
#6838=ORIENTED_EDGE('',*,*,#4924,.F.) ;
#6839=ORIENTED_EDGE('',*,*,#4921,.T.) ;
#6840=ORIENTED_EDGE('',*,*,#4923,.T.) ;
#6841=ORIENTED_EDGE('',*,*,#4856,.F.) ;
#6842=ORIENTED_EDGE('',*,*,#4925,.T.) ;
#7676=PLANE('',#9448) ;
#7677=PLANE('',#9513) ;
#8042=ADVANCED_FACE('',(#1655),#237,.T.) ;
#8043=ADVANCED_FACE('',(#1656),#238,.T.) ;
#8044=ADVANCED_FACE('',(#1657),#239,.T.) ;
#8045=ADVANCED_FACE('',(#1658),#240,.T.) ;
#8046=ADVANCED_FACE('',(#1659),#241,.T.) ;
#8047=ADVANCED_FACE('',(#1660),#242,.T.) ;
#8048=ADVANCED_FACE('',(#1661),#243,.T.) ;
#8049=ADVANCED_FACE('',(#1662),#244,.T.) ;
#8050=ADVANCED_FACE('',(#1663),#245,.T.) ;
#8051=ADVANCED_FACE('',(#1664),#246,.T.) ;
#8052=ADVANCED_FACE('',(#1665),#247,.T.) ;
#8053=ADVANCED_FACE('',(#1666),#248,.T.) ;
#8054=ADVANCED_FACE('',(#1667),#249,.T.) ;
#8055=ADVANCED_FACE('',(#1668),#250,.T.) ;
#8056=ADVANCED_FACE('',(#1669),#251,.T.) ;
#8057=ADVANCED_FACE('',(#1670),#252,.T.) ;
#8058=ADVANCED_FACE('',(#1671),#253,.T.) ;
#8059=ADVANCED_FACE('',(#1672),#254,.T.) ;
#8060=ADVANCED_FACE('',(#1673),#255,.T.) ;
#8061=ADVANCED_FACE('',(#1674),#256,.T.) ;
#8062=ADVANCED_FACE('',(#1675),#257,.T.) ;
#8063=ADVANCED_FACE('',(#1676),#258,.T.) ;
#8064=ADVANCED_FACE('',(#1677),#259,.T.) ;
#8065=ADVANCED_FACE('',(#1678),#732,.T.) ;
#8066=ADVANCED_FACE('',(#1679),#7676,.T.) ;
#8067=ADVANCED_FACE('',(#1680),#733,.T.) ;
#8068=ADVANCED_FACE('',(#1681),#734,.T.) ;
#8069=ADVANCED_FACE('',(#1682),#735,.T.) ;
#8070=ADVANCED_FACE('',(#1683),#736,.T.) ;
#8071=ADVANCED_FACE('',(#1684),#737,.T.) ;
#8072=ADVANCED_FACE('',(#1685),#738,.T.) ;
#8073=ADVANCED_FACE('',(#1686),#739,.T.) ;
#8074=ADVANCED_FACE('',(#1687),#740,.T.) ;
#8075=ADVANCED_FACE('',(#1688),#741,.T.) ;
#8076=ADVANCED_FACE('',(#1689),#742,.T.) ;
#8077=ADVANCED_FACE('',(#1690),#743,.T.) ;
#8078=ADVANCED_FACE('',(#1691),#744,.T.) ;
#8079=ADVANCED_FACE('',(#1692),#745,.T.) ;
#8080=ADVANCED_FACE('',(#1693),#746,.T.) ;
#8081=ADVANCED_FACE('',(#1694),#747,.T.) ;
#8082=ADVANCED_FACE('',(#1695),#748,.T.) ;
#8083=ADVANCED_FACE('',(#1696),#749,.T.) ;
#8084=ADVANCED_FACE('',(#1697),#750,.T.) ;
#8085=ADVANCED_FACE('',(#1698),#751,.T.) ;
#8086=ADVANCED_FACE('',(#1699),#752,.T.) ;
#8087=ADVANCED_FACE('',(#1700),#753,.T.) ;
#8088=ADVANCED_FACE('',(#1701),#754,.T.) ;
#8089=ADVANCED_FACE('',(#1702),#755,.T.) ;
#8090=ADVANCED_FACE('',(#1703),#7677,.T.) ;
#8274=CLOSED_SHELL('',(#8042,#8043,#8044,#8045,#8046,#8047,#8048,#8049,
#8050,#8051,#8052,#8053,#8054,#8055,#8056,#8057,#8058,#8059,#8060,#8061,
#8062,#8063,#8064,#8065,#8066,#8067,#8068,#8069,#8070,#8071,#8072,#8073,
#8074,#8075,#8076,#8077,#8078,#8079,#8080,#8081,#8082,#8083,#8084,#8085,
#8086,#8087,#8088,#8089,#8090)) ;
#9349=AXIS2_PLACEMENT_3D('',#14334,#11566,#11567) ;
#9350=AXIS2_PLACEMENT_3D('',#14335,#11568,#11569) ;
#9351=AXIS2_PLACEMENT_3D('',#14338,#11570,#11571) ;
#9352=AXIS2_PLACEMENT_3D('',#14339,#11572,#11573) ;
#9353=AXIS2_PLACEMENT_3D('',#14340,#11574,#11575) ;
#9354=AXIS2_PLACEMENT_3D('',#14343,#11576,#11577) ;
#9355=AXIS2_PLACEMENT_3D('',#14345,#11578,#11579) ;
#9356=AXIS2_PLACEMENT_3D('',#14346,#11580,#11581) ;
#9357=AXIS2_PLACEMENT_3D('',#14347,#11582,#11583) ;
#9358=AXIS2_PLACEMENT_3D('',#14350,#11584,#11585) ;
#9359=AXIS2_PLACEMENT_3D('',#14352,#11586,#11587) ;
#9360=AXIS2_PLACEMENT_3D('',#14354,#11588,#11589) ;
#9361=AXIS2_PLACEMENT_3D('',#14355,#11590,#11591) ;
#9362=AXIS2_PLACEMENT_3D('',#14356,#11592,#11593) ;
#9363=AXIS2_PLACEMENT_3D('',#14359,#11594,#11595) ;
#9364=AXIS2_PLACEMENT_3D('',#14361,#11596,#11597) ;
#9365=AXIS2_PLACEMENT_3D('',#14363,#11598,#11599) ;
#9366=AXIS2_PLACEMENT_3D('',#14364,#11600,#11601) ;
#9367=AXIS2_PLACEMENT_3D('',#14365,#11602,#11603) ;
#9368=AXIS2_PLACEMENT_3D('',#14368,#11604,#11605) ;
#9369=AXIS2_PLACEMENT_3D('',#14370,#11606,#11607) ;
#9370=AXIS2_PLACEMENT_3D('',#14372,#11608,#11609) ;
#9371=AXIS2_PLACEMENT_3D('',#14373,#11610,#11611) ;
#9372=AXIS2_PLACEMENT_3D('',#14374,#11612,#11613) ;
#9373=AXIS2_PLACEMENT_3D('',#14377,#11614,#11615) ;
#9374=AXIS2_PLACEMENT_3D('',#14379,#11616,#11617) ;
#9375=AXIS2_PLACEMENT_3D('',#14380,#11618,#11619) ;
#9376=AXIS2_PLACEMENT_3D('',#14381,#11620,#11621) ;
#9377=AXIS2_PLACEMENT_3D('',#14384,#11622,#11623) ;
#9378=AXIS2_PLACEMENT_3D('',#14385,#11624,#11625) ;
#9379=AXIS2_PLACEMENT_3D('',#14386,#11626,#11627) ;
#9380=AXIS2_PLACEMENT_3D('',#14389,#11628,#11629) ;
#9381=AXIS2_PLACEMENT_3D('',#14390,#11630,#11631) ;
#9382=AXIS2_PLACEMENT_3D('',#14391,#11632,#11633) ;
#9383=AXIS2_PLACEMENT_3D('',#14394,#11634,#11635) ;
#9384=AXIS2_PLACEMENT_3D('',#14395,#11636,#11637) ;
#9385=AXIS2_PLACEMENT_3D('',#14396,#11638,#11639) ;
#9386=AXIS2_PLACEMENT_3D('',#14399,#11640,#11641) ;
#9387=AXIS2_PLACEMENT_3D('',#14401,#11642,#11643) ;
#9388=AXIS2_PLACEMENT_3D('',#14402,#11644,#11645) ;
#9389=AXIS2_PLACEMENT_3D('',#14403,#11646,#11647) ;
#9390=AXIS2_PLACEMENT_3D('',#14406,#11648,#11649) ;
#9391=AXIS2_PLACEMENT_3D('',#14408,#11650,#11651) ;
#9392=AXIS2_PLACEMENT_3D('',#14410,#11652,#11653) ;
#9393=AXIS2_PLACEMENT_3D('',#14411,#11654,#11655) ;
#9394=AXIS2_PLACEMENT_3D('',#14412,#11656,#11657) ;
#9395=AXIS2_PLACEMENT_3D('',#14415,#11658,#11659) ;
#9396=AXIS2_PLACEMENT_3D('',#14417,#11660,#11661) ;
#9397=AXIS2_PLACEMENT_3D('',#14419,#11662,#11663) ;
#9398=AXIS2_PLACEMENT_3D('',#14420,#11664,#11665) ;
#9399=AXIS2_PLACEMENT_3D('',#14421,#11666,#11667) ;
#9400=AXIS2_PLACEMENT_3D('',#14424,#11668,#11669) ;
#9401=AXIS2_PLACEMENT_3D('',#14426,#11670,#11671) ;
#9402=AXIS2_PLACEMENT_3D('',#14428,#11672,#11673) ;
#9403=AXIS2_PLACEMENT_3D('',#14429,#11674,#11675) ;
#9404=AXIS2_PLACEMENT_3D('',#14430,#11676,#11677) ;
#9405=AXIS2_PLACEMENT_3D('',#14433,#11678,#11679) ;
#9406=AXIS2_PLACEMENT_3D('',#14435,#11680,#11681) ;
#9407=AXIS2_PLACEMENT_3D('',#14436,#11682,#11683) ;
#9408=AXIS2_PLACEMENT_3D('',#14437,#11684,#11685) ;
#9409=AXIS2_PLACEMENT_3D('',#14440,#11686,#11687) ;
#9410=AXIS2_PLACEMENT_3D('',#14441,#11688,#11689) ;
#9411=AXIS2_PLACEMENT_3D('',#14442,#11690,#11691) ;
#9412=AXIS2_PLACEMENT_3D('',#14445,#11692,#11693) ;
#9413=AXIS2_PLACEMENT_3D('',#14446,#11694,#11695) ;
#9414=AXIS2_PLACEMENT_3D('',#14447,#11696,#11697) ;
#9415=AXIS2_PLACEMENT_3D('',#14450,#11698,#11699) ;
#9416=AXIS2_PLACEMENT_3D('',#14451,#11700,#11701) ;
#9417=AXIS2_PLACEMENT_3D('',#14452,#11702,#11703) ;
#9418=AXIS2_PLACEMENT_3D('',#14455,#11704,#11705) ;
#9419=AXIS2_PLACEMENT_3D('',#14457,#11706,#11707) ;
#9420=AXIS2_PLACEMENT_3D('',#14458,#11708,#11709) ;
#9421=AXIS2_PLACEMENT_3D('',#14459,#11710,#11711) ;
#9422=AXIS2_PLACEMENT_3D('',#14462,#11712,#11713) ;
#9423=AXIS2_PLACEMENT_3D('',#14464,#11714,#11715) ;
#9424=AXIS2_PLACEMENT_3D('',#14466,#11716,#11717) ;
#9425=AXIS2_PLACEMENT_3D('',#14467,#11718,#11719) ;
#9426=AXIS2_PLACEMENT_3D('',#14468,#11720,#11721) ;
#9427=AXIS2_PLACEMENT_3D('',#14471,#11722,#11723) ;
#9428=AXIS2_PLACEMENT_3D('',#14473,#11724,#11725) ;
#9429=AXIS2_PLACEMENT_3D('',#14475,#11726,#11727) ;
#9430=AXIS2_PLACEMENT_3D('',#14476,#11728,#11729) ;
#9431=AXIS2_PLACEMENT_3D('',#14477,#11730,#11731) ;
#9432=AXIS2_PLACEMENT_3D('',#14480,#11732,#11733) ;
#9433=AXIS2_PLACEMENT_3D('',#14482,#11734,#11735) ;
#9434=AXIS2_PLACEMENT_3D('',#14484,#11736,#11737) ;
#9435=AXIS2_PLACEMENT_3D('',#14485,#11738,#11739) ;
#9436=AXIS2_PLACEMENT_3D('',#14486,#11740,#11741) ;
#9437=AXIS2_PLACEMENT_3D('',#14489,#11742,#11743) ;
#9438=AXIS2_PLACEMENT_3D('',#14491,#11744,#11745) ;
#9439=AXIS2_PLACEMENT_3D('',#14492,#11746,#11747) ;
#9440=AXIS2_PLACEMENT_3D('',#14493,#11748,#11749) ;
#9441=AXIS2_PLACEMENT_3D('',#14496,#11750,#11751) ;
#9442=AXIS2_PLACEMENT_3D('',#14497,#11752,#11753) ;
#9443=AXIS2_PLACEMENT_3D('',#14498,#11754,#11755) ;
#9444=AXIS2_PLACEMENT_3D('',#14500,#11756,#11757) ;
#9445=AXIS2_PLACEMENT_3D('',#14504,#11759,#11760) ;
#9446=AXIS2_PLACEMENT_3D('',#14505,#11761,#11762) ;
#9447=AXIS2_PLACEMENT_3D('',#14506,#11763,#11764) ;
#9448=AXIS2_PLACEMENT_3D('',#14507,#11765,#11766) ;
#9449=AXIS2_PLACEMENT_3D('',#14508,#11767,#11768) ;
#9450=AXIS2_PLACEMENT_3D('',#14511,#11770,#11771) ;
#9451=AXIS2_PLACEMENT_3D('',#14512,#11772,#11773) ;
#9452=AXIS2_PLACEMENT_3D('',#14513,#11774,#11775) ;
#9453=AXIS2_PLACEMENT_3D('',#14515,#11777,#11778) ;
#9454=AXIS2_PLACEMENT_3D('',#14516,#11779,#11780) ;
#9455=AXIS2_PLACEMENT_3D('',#14518,#11782,#11783) ;
#9456=AXIS2_PLACEMENT_3D('',#14519,#11784,#11785) ;
#9457=AXIS2_PLACEMENT_3D('',#14521,#11787,#11788) ;
#9458=AXIS2_PLACEMENT_3D('',#14522,#11789,#11790) ;
#9459=AXIS2_PLACEMENT_3D('',#14525,#11792,#11793) ;
#9460=AXIS2_PLACEMENT_3D('',#14526,#11794,#11795) ;
#9461=AXIS2_PLACEMENT_3D('',#14527,#11796,#11797) ;
#9462=AXIS2_PLACEMENT_3D('',#14531,#11799,#11800) ;
#9463=AXIS2_PLACEMENT_3D('',#14532,#11801,#11802) ;
#9464=AXIS2_PLACEMENT_3D('',#14533,#11803,#11804) ;
#9465=AXIS2_PLACEMENT_3D('',#14534,#11805,#11806) ;
#9466=AXIS2_PLACEMENT_3D('',#14537,#11808,#11809) ;
#9467=AXIS2_PLACEMENT_3D('',#14538,#11810,#11811) ;
#9468=AXIS2_PLACEMENT_3D('',#14539,#11812,#11813) ;
#9469=AXIS2_PLACEMENT_3D('',#14543,#11815,#11816) ;
#9470=AXIS2_PLACEMENT_3D('',#14544,#11817,#11818) ;
#9471=AXIS2_PLACEMENT_3D('',#14545,#11819,#11820) ;
#9472=AXIS2_PLACEMENT_3D('',#14546,#11821,#11822) ;
#9473=AXIS2_PLACEMENT_3D('',#14549,#11824,#11825) ;
#9474=AXIS2_PLACEMENT_3D('',#14550,#11826,#11827) ;
#9475=AXIS2_PLACEMENT_3D('',#14551,#11828,#11829) ;
#9476=AXIS2_PLACEMENT_3D('',#14553,#11831,#11832) ;
#9477=AXIS2_PLACEMENT_3D('',#14554,#11833,#11834) ;
#9478=AXIS2_PLACEMENT_3D('',#14556,#11836,#11837) ;
#9479=AXIS2_PLACEMENT_3D('',#14557,#11838,#11839) ;
#9480=AXIS2_PLACEMENT_3D('',#14559,#11841,#11842) ;
#9481=AXIS2_PLACEMENT_3D('',#14560,#11843,#11844) ;
#9482=AXIS2_PLACEMENT_3D('',#14563,#11846,#11847) ;
#9483=AXIS2_PLACEMENT_3D('',#14564,#11848,#11849) ;
#9484=AXIS2_PLACEMENT_3D('',#14565,#11850,#11851) ;
#9485=AXIS2_PLACEMENT_3D('',#14569,#11853,#11854) ;
#9486=AXIS2_PLACEMENT_3D('',#14570,#11855,#11856) ;
#9487=AXIS2_PLACEMENT_3D('',#14571,#11857,#11858) ;
#9488=AXIS2_PLACEMENT_3D('',#14572,#11859,#11860) ;
#9489=AXIS2_PLACEMENT_3D('',#14575,#11862,#11863) ;
#9490=AXIS2_PLACEMENT_3D('',#14576,#11864,#11865) ;
#9491=AXIS2_PLACEMENT_3D('',#14577,#11866,#11867) ;
#9492=AXIS2_PLACEMENT_3D('',#14581,#11869,#11870) ;
#9493=AXIS2_PLACEMENT_3D('',#14582,#11871,#11872) ;
#9494=AXIS2_PLACEMENT_3D('',#14583,#11873,#11874) ;
#9495=AXIS2_PLACEMENT_3D('',#14584,#11875,#11876) ;
#9496=AXIS2_PLACEMENT_3D('',#14587,#11878,#11879) ;
#9497=AXIS2_PLACEMENT_3D('',#14588,#11880,#11881) ;
#9498=AXIS2_PLACEMENT_3D('',#14589,#11882,#11883) ;
#9499=AXIS2_PLACEMENT_3D('',#14591,#11885,#11886) ;
#9500=AXIS2_PLACEMENT_3D('',#14592,#11887,#11888) ;
#9501=AXIS2_PLACEMENT_3D('',#14594,#11890,#11891) ;
#9502=AXIS2_PLACEMENT_3D('',#14595,#11892,#11893) ;
#9503=AXIS2_PLACEMENT_3D('',#14597,#11895,#11896) ;
#9504=AXIS2_PLACEMENT_3D('',#14598,#11897,#11898) ;
#9505=AXIS2_PLACEMENT_3D('',#14601,#11900,#11901) ;
#9506=AXIS2_PLACEMENT_3D('',#14602,#11902,#11903) ;
#9507=AXIS2_PLACEMENT_3D('',#14603,#11904,#11905) ;
#9508=AXIS2_PLACEMENT_3D('',#14607,#11907,#11908) ;
#9509=AXIS2_PLACEMENT_3D('',#14608,#11909,#11910) ;
#9510=AXIS2_PLACEMENT_3D('',#14609,#11911,#11912) ;
#9511=AXIS2_PLACEMENT_3D('',#14610,#11913,#11914) ;
#9512=AXIS2_PLACEMENT_3D('',#14613,#11916,#11917) ;
#9513=AXIS2_PLACEMENT_3D('',#14614,#11918,#11919) ;
#11566=DIRECTION('axis',(0.,0.,1.)) ;
#11567=DIRECTION('refdir',(1.,0.,0.)) ;
#11568=DIRECTION('center_axis',(0.,0.,1.)) ;
#11569=DIRECTION('ref_axis',(1.,0.,0.)) ;
#11570=DIRECTION('center_axis',(-0.381576765574098,-0.921207802535445,-0.0759957664730569)) ;
#11571=DIRECTION('ref_axis',(0.924337152760836,-0.38028493462931,-0.0313719065402714)) ;
#11572=DIRECTION('center_axis',(0.921207802535446,0.381576765574096,0.0759957664730549)) ;
#11573=DIRECTION('ref_axis',(0.389070924829671,-0.90346379356664,-0.179936069664646)) ;
#11574=DIRECTION('center_axis',(0.,0.,1.)) ;
#11575=DIRECTION('ref_axis',(1.,0.,0.)) ;
#11576=DIRECTION('center_axis',(-0.921207802535446,-0.381576765574096,-0.0759957664730549)) ;
#11577=DIRECTION('ref_axis',(0.389070924829671,-0.90346379356664,-0.179936069664646)) ;
#11578=DIRECTION('center_axis',(0.921207802535444,-0.381576765574099,0.075995766473057)) ;
#11579=DIRECTION('ref_axis',(0.389070924829674,0.903463793566638,-0.179936069664649)) ;
#11580=DIRECTION('center_axis',(0.921207802535444,-0.381576765574099,0.075995766473057)) ;
#11581=DIRECTION('ref_axis',(0.389070924829674,0.903463793566638,-0.179936069664649)) ;
#11582=DIRECTION('center_axis',(0.,0.,1.)) ;
#11583=DIRECTION('ref_axis',(-0.707106781186494,-0.707106781186601,0.)) ;
#11584=DIRECTION('center_axis',(-0.921207802535444,0.381576765574099,-0.075995766473057)) ;
#11585=DIRECTION('ref_axis',(0.389070924829674,0.903463793566638,-0.179936069664649)) ;
#11586=DIRECTION('center_axis',(-0.921207802535444,0.381576765574099,-0.075995766473057)) ;
#11587=DIRECTION('ref_axis',(0.389070924829674,0.903463793566638,-0.179936069664649)) ;
#11588=DIRECTION('center_axis',(0.381576765574096,-0.921207802535445,0.0759957664730569)) ;
#11589=DIRECTION('ref_axis',(0.924337152760837,0.380284934629308,-0.0313719065402712)) ;
#11590=DIRECTION('center_axis',(0.381576765574096,-0.921207802535445,0.0759957664730569)) ;
#11591=DIRECTION('ref_axis',(0.924337152760837,0.380284934629308,-0.0313719065402712)) ;
#11592=DIRECTION('center_axis',(0.,0.,1.)) ;
#11593=DIRECTION('ref_axis',(-1.,0.,0.)) ;
#11594=DIRECTION('center_axis',(-0.381576765574096,0.921207802535445,-0.0759957664730569)) ;
#11595=DIRECTION('ref_axis',(0.924337152760837,0.380284934629308,-0.0313719065402712)) ;
#11596=DIRECTION('center_axis',(-0.381576765574096,0.921207802535445,-0.0759957664730569)) ;
#11597=DIRECTION('ref_axis',(0.924337152760837,0.380284934629308,-0.0313719065402712)) ;
#11598=DIRECTION('center_axis',(-0.3815767655741,-0.921207802535444,0.0759957664730569)) ;
#11599=DIRECTION('ref_axis',(0.924337152760836,-0.380284934629312,0.0313719065402716)) ;
#11600=DIRECTION('center_axis',(-0.3815767655741,-0.921207802535444,0.0759957664730569)) ;
#11601=DIRECTION('ref_axis',(0.924337152760836,-0.380284934629312,0.0313719065402716)) ;
#11602=DIRECTION('center_axis',(0.,0.,1.)) ;
#11603=DIRECTION('ref_axis',(-0.707106781186548,0.707106781186548,0.)) ;
#11604=DIRECTION('center_axis',(0.3815767655741,0.921207802535444,-0.0759957664730569)) ;
#11605=DIRECTION('ref_axis',(0.924337152760836,-0.380284934629312,0.0313719065402716)) ;
#11606=DIRECTION('center_axis',(0.3815767655741,0.921207802535444,-0.0759957664730569)) ;
#11607=DIRECTION('ref_axis',(0.924337152760836,-0.380284934629312,0.0313719065402716)) ;
#11608=DIRECTION('center_axis',(-0.921207802535445,-0.381576765574097,0.0759957664730571)) ;
#11609=DIRECTION('ref_axis',(0.389070924829673,-0.903463793566638,0.17993606966465)) ;
#11610=DIRECTION('center_axis',(-0.921207802535445,-0.381576765574097,0.0759957664730571)) ;
#11611=DIRECTION('ref_axis',(0.389070924829673,-0.903463793566638,0.17993606966465)) ;
#11612=DIRECTION('center_axis',(0.,0.,1.)) ;
#11613=DIRECTION('ref_axis',(1.,0.,0.)) ;
#11614=DIRECTION('center_axis',(0.921207802535445,0.381576765574097,-0.0759957664730571)) ;
#11615=DIRECTION('ref_axis',(0.389070924829673,-0.903463793566638,0.17993606966465)) ;
#11616=DIRECTION('center_axis',(0.921207802535445,0.381576765574097,-0.0759957664730571)) ;
#11617=DIRECTION('ref_axis',(0.389070924829673,-0.903463793566638,0.17993606966465)) ;
#11618=DIRECTION('center_axis',(-0.921207802535444,0.381576765574099,0.075995766473057)) ;
#11619=DIRECTION('ref_axis',(0.389070924829674,0.903463793566638,0.179936069664649)) ;
#11620=DIRECTION('center_axis',(0.,0.,1.)) ;
#11621=DIRECTION('ref_axis',(1.,0.,0.)) ;
#11622=DIRECTION('center_axis',(0.921207802535444,-0.381576765574099,-0.075995766473057)) ;
#11623=DIRECTION('ref_axis',(0.389070924829674,0.903463793566638,0.179936069664649)) ;
#11624=DIRECTION('center_axis',(-0.381576765574098,0.921207802535444,0.075995766473057)) ;
#11625=DIRECTION('ref_axis',(0.924337152760836,0.380284934629311,0.0313719065402715)) ;
#11626=DIRECTION('center_axis',(0.,0.,1.)) ;
#11627=DIRECTION('ref_axis',(1.,0.,0.)) ;
#11628=DIRECTION('center_axis',(0.381576765574098,-0.921207802535444,-0.075995766473057)) ;
#11629=DIRECTION('ref_axis',(0.924337152760836,0.380284934629311,0.0313719065402715)) ;
#11630=DIRECTION('center_axis',(0.381576765574098,0.921207802535445,0.0759957664730568)) ;
#11631=DIRECTION('ref_axis',(0.924337152760837,-0.38028493462931,-0.0313719065402713)) ;
#11632=DIRECTION('center_axis',(0.,0.,1.)) ;
#11633=DIRECTION('ref_axis',(1.,0.,0.)) ;
#11634=DIRECTION('center_axis',(-0.381576765574098,-0.921207802535445,-0.0759957664730568)) ;
#11635=DIRECTION('ref_axis',(0.924337152760837,-0.38028493462931,-0.0313719065402713)) ;
#11636=DIRECTION('center_axis',(0.921207802535445,0.381576765574097,0.0759957664730571)) ;
#11637=DIRECTION('ref_axis',(0.389070924829673,-0.903463793566638,-0.17993606966465)) ;
#11638=DIRECTION('center_axis',(0.,0.,1.)) ;
#11639=DIRECTION('ref_axis',(1.,0.,0.)) ;
#11640=DIRECTION('center_axis',(-0.921207802535445,-0.381576765574097,-0.0759957664730571)) ;
#11641=DIRECTION('ref_axis',(0.389070924829673,-0.903463793566638,-0.17993606966465)) ;
#11642=DIRECTION('center_axis',(0.921207802535445,-0.381576765574097,0.0759957664730568)) ;
#11643=DIRECTION('ref_axis',(0.389070924829672,0.903463793566639,-0.179936069664649)) ;
#11644=DIRECTION('center_axis',(0.921207802535445,-0.381576765574097,0.0759957664730568)) ;
#11645=DIRECTION('ref_axis',(0.389070924829672,0.903463793566639,-0.179936069664649)) ;
#11646=DIRECTION('center_axis',(0.,0.,1.)) ;
#11647=DIRECTION('ref_axis',(-0.707106781186525,-0.70710678118657,0.)) ;
#11648=DIRECTION('center_axis',(-0.921207802535445,0.381576765574097,-0.0759957664730568)) ;
#11649=DIRECTION('ref_axis',(0.389070924829672,0.903463793566639,-0.179936069664649)) ;
#11650=DIRECTION('center_axis',(-0.921207802535445,0.381576765574097,-0.0759957664730568)) ;
#11651=DIRECTION('ref_axis',(0.389070924829672,0.903463793566639,-0.179936069664649)) ;
#11652=DIRECTION('center_axis',(0.381576765574097,-0.921207802535445,0.075995766473055)) ;
#11653=DIRECTION('ref_axis',(0.924337152760837,0.380284934629309,-0.0313719065402705)) ;
#11654=DIRECTION('center_axis',(0.381576765574097,-0.921207802535445,0.075995766473055)) ;
#11655=DIRECTION('ref_axis',(0.924337152760837,0.380284934629309,-0.0313719065402705)) ;
#11656=DIRECTION('center_axis',(0.,0.,1.)) ;
#11657=DIRECTION('ref_axis',(-1.,1.06581410364015E-13,0.)) ;
#11658=DIRECTION('center_axis',(-0.381576765574097,0.921207802535445,-0.075995766473055)) ;
#11659=DIRECTION('ref_axis',(0.924337152760837,0.380284934629309,-0.0313719065402705)) ;
#11660=DIRECTION('center_axis',(-0.381576765574097,0.921207802535445,-0.075995766473055)) ;
#11661=DIRECTION('ref_axis',(0.924337152760837,0.380284934629309,-0.0313719065402705)) ;
#11662=DIRECTION('center_axis',(-0.381576765574099,-0.921207802535444,0.0759957664730568)) ;
#11663=DIRECTION('ref_axis',(0.924337152760836,-0.380284934629311,0.0313719065402715)) ;
#11664=DIRECTION('center_axis',(-0.381576765574099,-0.921207802535444,0.0759957664730568)) ;
#11665=DIRECTION('ref_axis',(0.924337152760836,-0.380284934629311,0.0313719065402715)) ;
#11666=DIRECTION('center_axis',(0.,0.,1.)) ;
#11667=DIRECTION('ref_axis',(-0.707106781186494,0.707106781186601,0.)) ;
#11668=DIRECTION('center_axis',(0.381576765574099,0.921207802535444,-0.0759957664730568)) ;
#11669=DIRECTION('ref_axis',(0.924337152760836,-0.380284934629311,0.0313719065402715)) ;
#11670=DIRECTION('center_axis',(0.381576765574099,0.921207802535444,-0.0759957664730568)) ;
#11671=DIRECTION('ref_axis',(0.924337152760836,-0.380284934629311,0.0313719065402715)) ;
#11672=DIRECTION('center_axis',(-0.921207802535445,-0.381576765574097,0.0759957664730571)) ;
#11673=DIRECTION('ref_axis',(0.389070924829673,-0.903463793566638,0.17993606966465)) ;
#11674=DIRECTION('center_axis',(-0.921207802535445,-0.381576765574097,0.0759957664730571)) ;
#11675=DIRECTION('ref_axis',(0.389070924829673,-0.903463793566638,0.17993606966465)) ;
#11676=DIRECTION('center_axis',(0.,0.,1.)) ;
#11677=DIRECTION('ref_axis',(1.,0.,0.)) ;
#11678=DIRECTION('center_axis',(0.921207802535445,0.381576765574097,-0.0759957664730571)) ;
#11679=DIRECTION('ref_axis',(0.389070924829673,-0.903463793566638,0.17993606966465)) ;
#11680=DIRECTION('center_axis',(0.921207802535445,0.381576765574097,-0.0759957664730571)) ;
#11681=DIRECTION('ref_axis',(0.389070924829673,-0.903463793566638,0.17993606966465)) ;
#11682=DIRECTION('center_axis',(-0.921207802535444,0.381576765574099,0.075995766473057)) ;
#11683=DIRECTION('ref_axis',(0.389070924829674,0.903463793566638,0.179936069664649)) ;
#11684=DIRECTION('center_axis',(0.,0.,1.)) ;
#11685=DIRECTION('ref_axis',(1.,0.,0.)) ;
#11686=DIRECTION('center_axis',(0.921207802535444,-0.381576765574099,-0.075995766473057)) ;
#11687=DIRECTION('ref_axis',(0.389070924829674,0.903463793566638,0.179936069664649)) ;
#11688=DIRECTION('center_axis',(-0.381576765574098,0.921207802535444,0.075995766473057)) ;
#11689=DIRECTION('ref_axis',(0.924337152760836,0.380284934629311,0.0313719065402715)) ;
#11690=DIRECTION('center_axis',(0.,0.,1.)) ;
#11691=DIRECTION('ref_axis',(1.,0.,0.)) ;
#11692=DIRECTION('center_axis',(0.381576765574098,-0.921207802535444,-0.075995766473057)) ;
#11693=DIRECTION('ref_axis',(0.924337152760836,0.380284934629311,0.0313719065402715)) ;
#11694=DIRECTION('center_axis',(0.381576765574099,0.921207802535444,0.075995766473055)) ;
#11695=DIRECTION('ref_axis',(0.924337152760836,-0.380284934629311,-0.0313719065402707)) ;
#11696=DIRECTION('center_axis',(0.,0.,1.)) ;
#11697=DIRECTION('ref_axis',(1.,0.,0.)) ;
#11698=DIRECTION('center_axis',(-0.381576765574099,-0.921207802535444,-0.075995766473055)) ;
#11699=DIRECTION('ref_axis',(0.924337152760836,-0.380284934629311,-0.0313719065402707)) ;
#11700=DIRECTION('center_axis',(0.921207802535444,0.381576765574099,0.075995766473057)) ;
#11701=DIRECTION('ref_axis',(0.389070924829674,-0.903463793566638,-0.179936069664649)) ;
#11702=DIRECTION('center_axis',(0.,0.,1.)) ;
#11703=DIRECTION('ref_axis',(1.,0.,0.)) ;
#11704=DIRECTION('center_axis',(-0.921207802535444,-0.381576765574099,-0.075995766473057)) ;
#11705=DIRECTION('ref_axis',(0.389070924829674,-0.903463793566638,-0.179936069664649)) ;
#11706=DIRECTION('center_axis',(0.921207802535445,-0.381576765574097,0.0759957664730568)) ;
#11707=DIRECTION('ref_axis',(0.389070924829673,0.903463793566639,-0.179936069664649)) ;
#11708=DIRECTION('center_axis',(0.921207802535445,-0.381576765574097,0.0759957664730568)) ;
#11709=DIRECTION('ref_axis',(0.389070924829673,0.903463793566639,-0.179936069664649)) ;
#11710=DIRECTION('center_axis',(0.,0.,1.)) ;
#11711=DIRECTION('ref_axis',(-0.707106781186632,-0.707106781186463,0.)) ;
#11712=DIRECTION('center_axis',(-0.921207802535445,0.381576765574097,-0.0759957664730568)) ;
#11713=DIRECTION('ref_axis',(0.389070924829673,0.903463793566639,-0.179936069664649)) ;
#11714=DIRECTION('center_axis',(-0.921207802535445,0.381576765574097,-0.0759957664730568)) ;
#11715=DIRECTION('ref_axis',(0.389070924829673,0.903463793566639,-0.179936069664649)) ;
#11716=DIRECTION('center_axis',(0.381576765574097,-0.921207802535445,0.075995766473057)) ;
#11717=DIRECTION('ref_axis',(0.924337152760837,0.380284934629309,-0.0313719065402713)) ;
#11718=DIRECTION('center_axis',(0.381576765574097,-0.921207802535445,0.075995766473057)) ;
#11719=DIRECTION('ref_axis',(0.924337152760837,0.380284934629309,-0.0313719065402713)) ;
#11720=DIRECTION('center_axis',(0.,0.,1.)) ;
#11721=DIRECTION('ref_axis',(-1.,0.,0.)) ;
#11722=DIRECTION('center_axis',(-0.381576765574097,0.921207802535445,-0.075995766473057)) ;
#11723=DIRECTION('ref_axis',(0.924337152760837,0.380284934629309,-0.0313719065402713)) ;
#11724=DIRECTION('center_axis',(-0.381576765574097,0.921207802535445,-0.075995766473057)) ;
#11725=DIRECTION('ref_axis',(0.924337152760837,0.380284934629309,-0.0313719065402713)) ;
#11726=DIRECTION('center_axis',(-0.381576765574097,-0.921207802535445,0.075995766473057)) ;
#11727=DIRECTION('ref_axis',(0.924337152760837,-0.380284934629309,0.0313719065402713)) ;
#11728=DIRECTION('center_axis',(-0.381576765574097,-0.921207802535445,0.075995766473057)) ;
#11729=DIRECTION('ref_axis',(0.924337152760837,-0.380284934629309,0.0313719065402713)) ;
#11730=DIRECTION('center_axis',(0.,0.,1.)) ;
#11731=DIRECTION('ref_axis',(-0.707106781186601,0.707106781186494,0.)) ;
#11732=DIRECTION('center_axis',(0.381576765574097,0.921207802535445,-0.075995766473057)) ;
#11733=DIRECTION('ref_axis',(0.924337152760837,-0.380284934629309,0.0313719065402713)) ;
#11734=DIRECTION('center_axis',(0.381576765574097,0.921207802535445,-0.075995766473057)) ;
#11735=DIRECTION('ref_axis',(0.924337152760837,-0.380284934629309,0.0313719065402713)) ;
#11736=DIRECTION('center_axis',(-0.921207802535445,-0.381576765574098,0.0759957664730548)) ;
#11737=DIRECTION('ref_axis',(0.389070924829673,-0.90346379356664,0.179936069664645)) ;
#11738=DIRECTION('center_axis',(-0.921207802535445,-0.381576765574098,0.0759957664730548)) ;
#11739=DIRECTION('ref_axis',(0.389070924829673,-0.90346379356664,0.179936069664645)) ;
#11740=DIRECTION('center_axis',(0.,0.,1.)) ;
#11741=DIRECTION('ref_axis',(1.,0.,0.)) ;
#11742=DIRECTION('center_axis',(0.921207802535445,0.381576765574098,-0.0759957664730548)) ;
#11743=DIRECTION('ref_axis',(0.389070924829673,-0.90346379356664,0.179936069664645)) ;
#11744=DIRECTION('center_axis',(0.921207802535445,0.381576765574098,-0.0759957664730548)) ;
#11745=DIRECTION('ref_axis',(0.389070924829673,-0.90346379356664,0.179936069664645)) ;
#11746=DIRECTION('center_axis',(-0.921207802535444,0.381576765574099,0.075995766473057)) ;
#11747=DIRECTION('ref_axis',(0.389070924829674,0.903463793566638,0.179936069664649)) ;
#11748=DIRECTION('center_axis',(0.,0.,1.)) ;
#11749=DIRECTION('ref_axis',(1.,0.,0.)) ;
#11750=DIRECTION('center_axis',(0.921207802535444,-0.381576765574099,-0.075995766473057)) ;
#11751=DIRECTION('ref_axis',(0.389070924829674,0.903463793566638,0.179936069664649)) ;
#11752=DIRECTION('center_axis',(-0.381576765574098,0.921207802535444,0.075995766473057)) ;
#11753=DIRECTION('ref_axis',(0.924337152760836,0.380284934629311,0.0313719065402715)) ;
#11754=DIRECTION('center_axis',(0.381576765574098,0.921207802535445,0.0759957664730569)) ;
#11755=DIRECTION('ref_axis',(0.924337152760836,-0.38028493462931,-0.0313719065402714)) ;
#11756=DIRECTION('center_axis',(0.381576765574098,0.921207802535445,0.0759957664730569)) ;
#11757=DIRECTION('ref_axis',(0.924337152760836,-0.38028493462931,-0.0313719065402714)) ;
#11758=DIRECTION('',(-0.381576765574098,-0.921207802535444,-0.0759957664730569)) ;
#11759=DIRECTION('center_axis',(-0.704712865980969,-0.704712865980954,-0.0822165010311149)) ;
#11760=DIRECTION('ref_axis',(0.70710678118654,-0.707106781186555,5.23532745586745E-15)) ;
#11761=DIRECTION('center_axis',(-0.704712865980969,-0.704712865980954,-0.0822165010311149)) ;
#11762=DIRECTION('ref_axis',(0.70710678118654,-0.707106781186555,5.23532745586745E-15)) ;
#11763=DIRECTION('center_axis',(-0.704712865980969,-0.704712865980954,-0.0822165010311149)) ;
#11764=DIRECTION('ref_axis',(0.70710678118654,-0.707106781186555,5.23532745586745E-15)) ;
#11765=DIRECTION('center_axis',(0.381576765574098,0.921207802535445,0.0759957664730569)) ;
#11766=DIRECTION('ref_axis',(0.924337152760836,-0.38028493462931,-0.0313719065402714)) ;
#11767=DIRECTION('center_axis',(0.921207802535446,0.381576765574096,0.0759957664730549)) ;
#11768=DIRECTION('ref_axis',(0.389070924829671,-0.90346379356664,-0.179936069664646)) ;
#11769=DIRECTION('',(-0.921207802535446,-0.381576765574096,-0.0759957664730549)) ;
#11770=DIRECTION('center_axis',(-0.996614492649089,-1.90638497962248E-14,
-0.0822165010311158)) ;
#11771=DIRECTION('ref_axis',(1.78786833485215E-14,-1.,1.54574446170177E-14)) ;
#11772=DIRECTION('center_axis',(-0.996614492649089,-1.90638497962248E-14,
-0.0822165010311158)) ;
#11773=DIRECTION('ref_axis',(1.78786833485215E-14,-1.,1.54574446170177E-14)) ;
#11774=DIRECTION('center_axis',(0.921207802535444,-0.381576765574099,0.075995766473057)) ;
#11775=DIRECTION('ref_axis',(0.389070924829674,0.903463793566638,-0.179936069664649)) ;
#11776=DIRECTION('',(-0.921207802535444,0.381576765574099,-0.075995766473057)) ;
#11777=DIRECTION('center_axis',(-0.704712865980983,0.70471286598094,-0.0822165010311149)) ;
#11778=DIRECTION('ref_axis',(0.707106781186526,0.707106781186569,-7.7287223085089E-15)) ;
#11779=DIRECTION('center_axis',(0.381576765574096,-0.921207802535445,0.0759957664730569)) ;
#11780=DIRECTION('ref_axis',(0.924337152760837,0.380284934629308,-0.0313719065402712)) ;
#11781=DIRECTION('',(-0.381576765574096,0.921207802535445,-0.0759957664730569)) ;
#11782=DIRECTION('center_axis',(8.18196890271355E-15,0.996614492649089,
-0.0822165010311158)) ;
#11783=DIRECTION('ref_axis',(1.,-8.08148556740336E-15,6.73457130616947E-16)) ;
#11784=DIRECTION('center_axis',(-0.3815767655741,-0.921207802535444,0.0759957664730569)) ;
#11785=DIRECTION('ref_axis',(0.924337152760836,-0.380284934629312,0.0313719065402716)) ;
#11786=DIRECTION('',(0.3815767655741,0.921207802535444,-0.0759957664730569)) ;
#11787=DIRECTION('center_axis',(0.704712865980961,0.704712865980961,-0.0822165010311149)) ;
#11788=DIRECTION('ref_axis',(0.707106781186547,-0.707106781186548,-5.99697540120808E-15)) ;
#11789=DIRECTION('center_axis',(-0.921207802535445,-0.381576765574097,0.0759957664730571)) ;
#11790=DIRECTION('ref_axis',(0.389070924829673,-0.903463793566638,0.17993606966465)) ;
#11791=DIRECTION('',(0.921207802535445,0.381576765574097,-0.0759957664730571)) ;
#11792=DIRECTION('center_axis',(0.996614492649089,1.34995599539884E-15,
-0.0822165010311158)) ;
#11793=DIRECTION('ref_axis',(7.0352218109092E-16,-1.,-7.98527740588669E-15)) ;
#11794=DIRECTION('center_axis',(0.996614492649089,1.34995599539884E-15,
-0.0822165010311158)) ;
#11795=DIRECTION('ref_axis',(7.0352218109092E-16,-1.,-7.98527740588669E-15)) ;
#11796=DIRECTION('center_axis',(-0.921207802535444,0.381576765574099,0.075995766473057)) ;
#11797=DIRECTION('ref_axis',(0.389070924829674,0.903463793566638,0.179936069664649)) ;
#11798=DIRECTION('',(0.921207802535444,-0.381576765574099,-0.075995766473057)) ;
#11799=DIRECTION('center_axis',(0.704712865980961,-0.704712865980961,-0.0822165010311149)) ;
#11800=DIRECTION('ref_axis',(0.707106781186548,0.707106781186547,5.35558765776336E-15)) ;
#11801=DIRECTION('center_axis',(0.704712865980961,-0.704712865980961,-0.0822165010311149)) ;
#11802=DIRECTION('ref_axis',(0.707106781186548,0.707106781186547,5.35558765776336E-15)) ;
#11803=DIRECTION('center_axis',(0.704712865980961,-0.704712865980961,-0.0822165010311149)) ;
#11804=DIRECTION('ref_axis',(0.707106781186548,0.707106781186547,5.35558765776336E-15)) ;
#11805=DIRECTION('center_axis',(-0.381576765574098,0.921207802535444,0.075995766473057)) ;
#11806=DIRECTION('ref_axis',(0.924337152760836,0.380284934629311,0.0313719065402715)) ;
#11807=DIRECTION('',(0.381576765574098,-0.921207802535444,-0.075995766473057)) ;
#11808=DIRECTION('center_axis',(0.,-0.996614492649089,-0.0822165010311158)) ;
#11809=DIRECTION('ref_axis',(1.,0.,4.00867339652946E-18)) ;
#11810=DIRECTION('center_axis',(0.,-0.996614492649089,-0.0822165010311158)) ;
#11811=DIRECTION('ref_axis',(1.,0.,4.00867339652946E-18)) ;
#11812=DIRECTION('center_axis',(0.381576765574098,0.921207802535445,0.0759957664730568)) ;
#11813=DIRECTION('ref_axis',(0.924337152760837,-0.38028493462931,-0.0313719065402713)) ;
#11814=DIRECTION('',(-0.381576765574098,-0.921207802535445,-0.0759957664730568)) ;
#11815=DIRECTION('center_axis',(-0.704712865980969,-0.704712865980953,-0.0822165010311149)) ;
#11816=DIRECTION('ref_axis',(0.707106781186539,-0.707106781186556,5.30748357700498E-15)) ;
#11817=DIRECTION('center_axis',(-0.704712865980969,-0.704712865980953,-0.0822165010311149)) ;
#11818=DIRECTION('ref_axis',(0.707106781186539,-0.707106781186556,5.30748357700498E-15)) ;
#11819=DIRECTION('center_axis',(-0.704712865980969,-0.704712865980953,-0.0822165010311149)) ;
#11820=DIRECTION('ref_axis',(0.707106781186539,-0.707106781186556,5.30748357700498E-15)) ;
#11821=DIRECTION('center_axis',(0.921207802535445,0.381576765574097,0.0759957664730571)) ;
#11822=DIRECTION('ref_axis',(0.389070924829673,-0.903463793566638,-0.17993606966465)) ;
#11823=DIRECTION('',(-0.921207802535445,-0.381576765574097,-0.0759957664730571)) ;
#11824=DIRECTION('center_axis',(-0.996614492649089,-1.34995599539884E-15,
-0.0822165010311158)) ;
#11825=DIRECTION('ref_axis',(7.0352218109092E-16,-1.,7.98527740588669E-15)) ;
#11826=DIRECTION('center_axis',(-0.996614492649089,-1.34995599539884E-15,
-0.0822165010311158)) ;
#11827=DIRECTION('ref_axis',(7.0352218109092E-16,-1.,7.98527740588669E-15)) ;
#11828=DIRECTION('center_axis',(0.921207802535445,-0.381576765574097,0.0759957664730568)) ;
#11829=DIRECTION('ref_axis',(0.389070924829672,0.903463793566639,-0.179936069664649)) ;
#11830=DIRECTION('',(-0.921207802535445,0.381576765574097,-0.0759957664730568)) ;
#11831=DIRECTION('center_axis',(-0.70471286598097,0.704712865980952,-0.0822165010311149)) ;
#11832=DIRECTION('ref_axis',(0.707106781186539,0.707106781186556,-6.87888354844459E-15)) ;
#11833=DIRECTION('center_axis',(0.381576765574097,-0.921207802535445,0.075995766473055)) ;
#11834=DIRECTION('ref_axis',(0.924337152760837,0.380284934629309,-0.0313719065402705)) ;
#11835=DIRECTION('',(-0.381576765574097,0.921207802535445,-0.075995766473055)) ;
#11836=DIRECTION('center_axis',(8.18196890271356E-15,0.99661449264909,-0.082216501031107)) ;
#11837=DIRECTION('ref_axis',(1.,-8.14562434174784E-15,6.73457130616947E-16)) ;
#11838=DIRECTION('center_axis',(-0.381576765574099,-0.921207802535444,0.0759957664730568)) ;
#11839=DIRECTION('ref_axis',(0.924337152760836,-0.380284934629311,0.0313719065402715)) ;
#11840=DIRECTION('',(0.381576765574099,0.921207802535444,-0.0759957664730568)) ;
#11841=DIRECTION('center_axis',(0.704712865980969,0.704712865980953,-0.0822165010311149)) ;
#11842=DIRECTION('ref_axis',(0.707106781186539,-0.707106781186556,-5.58007336796898E-15)) ;
#11843=DIRECTION('center_axis',(-0.921207802535445,-0.381576765574097,0.0759957664730571)) ;
#11844=DIRECTION('ref_axis',(0.389070924829673,-0.903463793566638,0.17993606966465)) ;
#11845=DIRECTION('',(0.921207802535445,0.381576765574097,-0.0759957664730571)) ;
#11846=DIRECTION('center_axis',(0.996614492649089,1.34995599539884E-15,
-0.0822165010311158)) ;
#11847=DIRECTION('ref_axis',(7.0352218109092E-16,-1.,-7.98527740588669E-15)) ;
#11848=DIRECTION('center_axis',(0.996614492649089,1.34995599539884E-15,
-0.0822165010311158)) ;
#11849=DIRECTION('ref_axis',(7.0352218109092E-16,-1.,-7.98527740588669E-15)) ;
#11850=DIRECTION('center_axis',(-0.921207802535444,0.381576765574099,0.075995766473057)) ;
#11851=DIRECTION('ref_axis',(0.389070924829674,0.903463793566638,0.179936069664649)) ;
#11852=DIRECTION('',(0.921207802535444,-0.381576765574099,-0.075995766473057)) ;
#11853=DIRECTION('center_axis',(0.704712865980961,-0.704712865980961,-0.0822165010311149)) ;
#11854=DIRECTION('ref_axis',(0.707106781186548,0.707106781186547,5.35558765776336E-15)) ;
#11855=DIRECTION('center_axis',(0.704712865980961,-0.704712865980961,-0.0822165010311149)) ;
#11856=DIRECTION('ref_axis',(0.707106781186548,0.707106781186547,5.35558765776336E-15)) ;
#11857=DIRECTION('center_axis',(0.704712865980961,-0.704712865980961,-0.0822165010311149)) ;
#11858=DIRECTION('ref_axis',(0.707106781186548,0.707106781186547,5.35558765776336E-15)) ;
#11859=DIRECTION('center_axis',(-0.381576765574098,0.921207802535444,0.075995766473057)) ;
#11860=DIRECTION('ref_axis',(0.924337152760836,0.380284934629311,0.0313719065402715)) ;
#11861=DIRECTION('',(0.381576765574098,-0.921207802535444,-0.075995766473057)) ;
#11862=DIRECTION('center_axis',(-6.83201290731471E-15,-0.996614492649089,
-0.0822165010311158)) ;
#11863=DIRECTION('ref_axis',(1.,-6.79871008051394E-15,-5.57205602117593E-16)) ;
#11864=DIRECTION('center_axis',(-6.83201290731471E-15,-0.996614492649089,
-0.0822165010311158)) ;
#11865=DIRECTION('ref_axis',(1.,-6.79871008051394E-15,-5.57205602117593E-16)) ;
#11866=DIRECTION('center_axis',(0.381576765574099,0.921207802535444,0.075995766473055)) ;
#11867=DIRECTION('ref_axis',(0.924337152760836,-0.380284934629311,-0.0313719065402707)) ;
#11868=DIRECTION('',(-0.381576765574099,-0.921207802535444,-0.075995766473055)) ;
#11869=DIRECTION('center_axis',(-0.704712865980962,-0.70471286598096,-0.0822165010311149)) ;
#11870=DIRECTION('ref_axis',(0.707106781186546,-0.707106781186549,1.06630712347684E-14)) ;
#11871=DIRECTION('center_axis',(-0.704712865980962,-0.70471286598096,-0.0822165010311149)) ;
#11872=DIRECTION('ref_axis',(0.707106781186546,-0.707106781186549,1.06630712347684E-14)) ;
#11873=DIRECTION('center_axis',(-0.704712865980962,-0.70471286598096,-0.0822165010311149)) ;
#11874=DIRECTION('ref_axis',(0.707106781186546,-0.707106781186549,1.06630712347684E-14)) ;
#11875=DIRECTION('center_axis',(0.921207802535444,0.381576765574099,0.075995766473057)) ;
#11876=DIRECTION('ref_axis',(0.389070924829674,-0.903463793566638,-0.179936069664649)) ;
#11877=DIRECTION('',(-0.921207802535444,-0.381576765574099,-0.075995766473057)) ;
#11878=DIRECTION('center_axis',(-0.996614492649089,-1.34995599539884E-15,
-0.0822165010311158)) ;
#11879=DIRECTION('ref_axis',(7.3759590496142E-16,-1.,8.33804066478127E-15)) ;
#11880=DIRECTION('center_axis',(-0.996614492649089,-1.34995599539884E-15,
-0.0822165010311158)) ;
#11881=DIRECTION('ref_axis',(7.3759590496142E-16,-1.,8.33804066478127E-15)) ;
#11882=DIRECTION('center_axis',(0.921207802535445,-0.381576765574097,0.0759957664730568)) ;
#11883=DIRECTION('ref_axis',(0.389070924829673,0.903463793566639,-0.179936069664649)) ;
#11884=DIRECTION('',(-0.921207802535445,0.381576765574097,-0.0759957664730568)) ;
#11885=DIRECTION('center_axis',(-0.704712865980969,0.704712865980953,-0.0822165010311149)) ;
#11886=DIRECTION('ref_axis',(0.70710678118654,0.707106781186555,-6.95905701637518E-15)) ;
#11887=DIRECTION('center_axis',(0.381576765574097,-0.921207802535445,0.075995766473057)) ;
#11888=DIRECTION('ref_axis',(0.924337152760837,0.380284934629309,-0.0313719065402713)) ;
#11889=DIRECTION('',(-0.381576765574097,0.921207802535445,-0.075995766473057)) ;
#11890=DIRECTION('center_axis',(0.,0.996614492649089,-0.0822165010311159)) ;
#11891=DIRECTION('ref_axis',(1.,0.,-4.00867339652946E-18)) ;
#11892=DIRECTION('center_axis',(-0.381576765574097,-0.921207802535445,0.075995766473057)) ;
#11893=DIRECTION('ref_axis',(0.924337152760837,-0.380284934629309,0.0313719065402713)) ;
#11894=DIRECTION('',(0.381576765574097,0.921207802535445,-0.075995766473057)) ;
#11895=DIRECTION('center_axis',(0.704712865980961,0.704712865980961,-0.0822165010311149)) ;
#11896=DIRECTION('ref_axis',(0.707106781186547,-0.707106781186548,-5.54800398079677E-15)) ;
#11897=DIRECTION('center_axis',(-0.921207802535445,-0.381576765574098,0.0759957664730548)) ;
#11898=DIRECTION('ref_axis',(0.389070924829673,-0.90346379356664,0.179936069664645)) ;
#11899=DIRECTION('',(0.921207802535445,0.381576765574098,-0.0759957664730548)) ;
#11900=DIRECTION('center_axis',(0.996614492649089,1.34995599539885E-15,
-0.0822165010311166)) ;
#11901=DIRECTION('ref_axis',(1.46316578973325E-16,-1.,-1.54895140041898E-14)) ;
#11902=DIRECTION('center_axis',(0.996614492649089,1.34995599539885E-15,
-0.0822165010311166)) ;
#11903=DIRECTION('ref_axis',(1.46316578973325E-16,-1.,-1.54895140041898E-14)) ;
#11904=DIRECTION('center_axis',(-0.921207802535444,0.381576765574099,0.075995766473057)) ;
#11905=DIRECTION('ref_axis',(0.389070924829674,0.903463793566638,0.179936069664649)) ;
#11906=DIRECTION('',(0.921207802535444,-0.381576765574099,-0.075995766473057)) ;
#11907=DIRECTION('center_axis',(0.704712865980961,-0.704712865980961,-0.0822165010311149)) ;
#11908=DIRECTION('ref_axis',(0.707106781186548,0.707106781186547,5.35558765776336E-15)) ;
#11909=DIRECTION('center_axis',(0.704712865980961,-0.704712865980961,-0.0822165010311149)) ;
#11910=DIRECTION('ref_axis',(0.707106781186548,0.707106781186547,5.35558765776336E-15)) ;
#11911=DIRECTION('center_axis',(0.704712865980961,-0.704712865980961,-0.0822165010311149)) ;
#11912=DIRECTION('ref_axis',(0.707106781186548,0.707106781186547,5.35558765776336E-15)) ;
#11913=DIRECTION('center_axis',(-0.381576765574098,0.921207802535444,0.075995766473057)) ;
#11914=DIRECTION('ref_axis',(0.924337152760836,0.380284934629311,0.0313719065402715)) ;
#11915=DIRECTION('',(0.381576765574098,-0.921207802535444,-0.075995766473057)) ;
#11916=DIRECTION('center_axis',(0.381576765574098,-0.921207802535444,-0.075995766473057)) ;
#11917=DIRECTION('ref_axis',(0.924337152760836,0.380284934629311,0.0313719065402715)) ;
#11918=DIRECTION('center_axis',(0.381576765574098,-0.921207802535444,-0.075995766473057)) ;
#11919=DIRECTION('ref_axis',(-0.924337152760836,-0.380284934629311,-0.0313719065402715)) ;
#14334=CARTESIAN_POINT('',(0.,0.,0.)) ;
#14335=CARTESIAN_POINT('Origin',(-2.78786796564404,1.58786796564404,2.3525)) ;
#14336=CARTESIAN_POINT('',(-2.78641456950892,1.58932136177915,2.32758463768377)) ;
#14337=CARTESIAN_POINT('',(-2.78932136177915,1.58641456950892,2.37741536231623)) ;
#14338=CARTESIAN_POINT('Origin',(-2.78786796564404,1.58786796564404,2.3525)) ;
#14339=CARTESIAN_POINT('Origin',(-2.78786796564404,1.58786796564404,2.3525)) ;
#14340=CARTESIAN_POINT('Origin',(-3.,1.5,2.335)) ;
#14341=CARTESIAN_POINT('',(-2.99794458747422,1.5,2.31008463768377)) ;
#14342=CARTESIAN_POINT('',(-3.00205541252578,1.5,2.35991536231623)) ;
#14343=CARTESIAN_POINT('Origin',(-3.,1.5,2.335)) ;
#14344=CARTESIAN_POINT('',(-3.00972677312074,1.47741340516083,2.33949840174162)) ;
#14345=CARTESIAN_POINT('Origin',(-3.,1.5,2.335)) ;
#14346=CARTESIAN_POINT('Origin',(-3.,1.5,2.335)) ;
#14347=CARTESIAN_POINT('Origin',(-3.21213203435596,1.58786796564404,2.3175)) ;
#14348=CARTESIAN_POINT('',(-3.21067863822085,1.58641456950892,2.29258463768377)) ;
#14349=CARTESIAN_POINT('',(-3.22185880747671,1.56528137080487,2.32199840174162)) ;
#14350=CARTESIAN_POINT('Origin',(-3.21213203435596,1.58786796564404,2.3175)) ;
#14351=CARTESIAN_POINT('',(-3.21358543049108,1.58932136177915,2.34241536231623)) ;
#14352=CARTESIAN_POINT('Origin',(-3.21213203435596,1.58786796564404,2.3175)) ;
#14353=CARTESIAN_POINT('',(-3.23524046317499,1.5783608422783,2.31828429766351)) ;
#14354=CARTESIAN_POINT('Origin',(-3.21213203435596,1.58786796564404,2.3175)) ;
#14355=CARTESIAN_POINT('Origin',(-3.21213203435596,1.58786796564404,2.3175)) ;
#14356=CARTESIAN_POINT('Origin',(-3.3,1.8,2.3)) ;
#14357=CARTESIAN_POINT('',(-3.3,1.79794458747422,2.27508463768377)) ;
#14358=CARTESIAN_POINT('',(-3.32310842881902,1.79049287663427,2.30078429766351)) ;
#14359=CARTESIAN_POINT('Origin',(-3.3,1.8,2.3)) ;
#14360=CARTESIAN_POINT('',(-3.3,1.80205541252578,2.32491536231623)) ;
#14361=CARTESIAN_POINT('Origin',(-3.3,1.8,2.3)) ;
#14362=CARTESIAN_POINT('',(-3.32310842881902,1.80950712336573,2.29921570233649)) ;
#14363=CARTESIAN_POINT('Origin',(-3.3,1.8,2.3)) ;
#14364=CARTESIAN_POINT('Origin',(-3.3,1.8,2.3)) ;
#14365=CARTESIAN_POINT('Origin',(-3.21213203435596,2.01213203435596,2.2825)) ;
#14366=CARTESIAN_POINT('',(-3.21358543049108,2.01067863822085,2.25758463768377)) ;
#14367=CARTESIAN_POINT('',(-3.23524046317498,2.0216391577217,2.28171570233649)) ;
#14368=CARTESIAN_POINT('Origin',(-3.21213203435596,2.01213203435596,2.2825)) ;
#14369=CARTESIAN_POINT('',(-3.21067863822085,2.01358543049108,2.30741536231623)) ;
#14370=CARTESIAN_POINT('Origin',(-3.21213203435596,2.01213203435596,2.2825)) ;
#14371=CARTESIAN_POINT('',(-3.22185880747671,2.03471862919513,2.27800159825838)) ;
#14372=CARTESIAN_POINT('Origin',(-3.21213203435596,2.01213203435596,2.2825)) ;
#14373=CARTESIAN_POINT('Origin',(-3.21213203435596,2.01213203435596,2.2825)) ;
#14374=CARTESIAN_POINT('Origin',(-3.,2.1,2.265)) ;
#14375=CARTESIAN_POINT('',(-3.00205541252578,2.1,2.24008463768377)) ;
#14376=CARTESIAN_POINT('',(-3.00972677312074,2.12258659483917,2.26050159825838)) ;
#14377=CARTESIAN_POINT('Origin',(-3.,2.1,2.265)) ;
#14378=CARTESIAN_POINT('',(-2.99794458747422,2.1,2.28991536231623)) ;
#14379=CARTESIAN_POINT('Origin',(-3.,2.1,2.265)) ;
#14380=CARTESIAN_POINT('Origin',(-3.,2.1,2.265)) ;
#14381=CARTESIAN_POINT('Origin',(-2.78786796564404,2.01213203435596,2.2475)) ;
#14382=CARTESIAN_POINT('',(-2.78932136177915,2.01358543049108,2.22258463768377)) ;
#14383=CARTESIAN_POINT('',(-2.78641456950892,2.01067863822085,2.27241536231623)) ;
#14384=CARTESIAN_POINT('Origin',(-2.78786796564404,2.01213203435596,2.2475)) ;
#14385=CARTESIAN_POINT('Origin',(-2.78786796564404,2.01213203435596,2.2475)) ;
#14386=CARTESIAN_POINT('Origin',(-2.7,1.8,2.23)) ;
#14387=CARTESIAN_POINT('',(-2.7,1.80205541252578,2.20508463768377)) ;
#14388=CARTESIAN_POINT('',(-2.7,1.79794458747422,2.25491536231623)) ;
#14389=CARTESIAN_POINT('Origin',(-2.7,1.8,2.23)) ;
#14390=CARTESIAN_POINT('Origin',(-2.7,1.8,2.23)) ;
#14391=CARTESIAN_POINT('Origin',(-2.78786796564404,1.58786796564404,2.2125)) ;
#14392=CARTESIAN_POINT('',(-2.78641456950892,1.58932136177915,2.18758463768377)) ;
#14393=CARTESIAN_POINT('',(-2.78932136177915,1.58641456950892,2.23741536231623)) ;
#14394=CARTESIAN_POINT('Origin',(-2.78786796564404,1.58786796564404,2.2125)) ;
#14395=CARTESIAN_POINT('Origin',(-2.78786796564404,1.58786796564404,2.2125)) ;
#14396=CARTESIAN_POINT('Origin',(-3.,1.5,2.195)) ;
#14397=CARTESIAN_POINT('',(-2.99794458747422,1.5,2.17008463768377)) ;
#14398=CARTESIAN_POINT('',(-3.00205541252578,1.5,2.21991536231623)) ;
#14399=CARTESIAN_POINT('Origin',(-3.,1.5,2.195)) ;
#14400=CARTESIAN_POINT('',(-3.00972677312074,1.47741340516083,2.19949840174162)) ;
#14401=CARTESIAN_POINT('Origin',(-3.,1.5,2.195)) ;
#14402=CARTESIAN_POINT('Origin',(-3.,1.5,2.195)) ;
#14403=CARTESIAN_POINT('Origin',(-3.21213203435596,1.58786796564404,2.1775)) ;
#14404=CARTESIAN_POINT('',(-3.21067863822085,1.58641456950892,2.15258463768377)) ;
#14405=CARTESIAN_POINT('',(-3.22185880747671,1.56528137080487,2.18199840174162)) ;
#14406=CARTESIAN_POINT('Origin',(-3.21213203435596,1.58786796564404,2.1775)) ;
#14407=CARTESIAN_POINT('',(-3.21358543049108,1.58932136177915,2.20241536231623)) ;
#14408=CARTESIAN_POINT('Origin',(-3.21213203435596,1.58786796564404,2.1775)) ;
#14409=CARTESIAN_POINT('',(-3.23524046317499,1.5783608422783,2.17828429766351)) ;
#14410=CARTESIAN_POINT('Origin',(-3.21213203435596,1.58786796564404,2.1775)) ;
#14411=CARTESIAN_POINT('Origin',(-3.21213203435596,1.58786796564404,2.1775)) ;
#14412=CARTESIAN_POINT('Origin',(-3.3,1.8,2.16)) ;
#14413=CARTESIAN_POINT('',(-3.3,1.79794458747422,2.13508463768377)) ;
#14414=CARTESIAN_POINT('',(-3.32310842881902,1.79049287663427,2.16078429766351)) ;
#14415=CARTESIAN_POINT('Origin',(-3.3,1.8,2.16)) ;
#14416=CARTESIAN_POINT('',(-3.3,1.80205541252578,2.18491536231623)) ;
#14417=CARTESIAN_POINT('Origin',(-3.3,1.8,2.16)) ;
#14418=CARTESIAN_POINT('',(-3.32310842881902,1.80950712336573,2.15921570233649)) ;
#14419=CARTESIAN_POINT('Origin',(-3.3,1.8,2.16)) ;
#14420=CARTESIAN_POINT('Origin',(-3.3,1.8,2.16)) ;
#14421=CARTESIAN_POINT('Origin',(-3.21213203435596,2.01213203435596,2.1425)) ;
#14422=CARTESIAN_POINT('',(-3.21358543049108,2.01067863822085,2.11758463768377)) ;
#14423=CARTESIAN_POINT('',(-3.23524046317498,2.0216391577217,2.14171570233649)) ;
#14424=CARTESIAN_POINT('Origin',(-3.21213203435596,2.01213203435596,2.1425)) ;
#14425=CARTESIAN_POINT('',(-3.21067863822085,2.01358543049108,2.16741536231623)) ;
#14426=CARTESIAN_POINT('Origin',(-3.21213203435596,2.01213203435596,2.1425)) ;
#14427=CARTESIAN_POINT('',(-3.22185880747671,2.03471862919513,2.13800159825838)) ;
#14428=CARTESIAN_POINT('Origin',(-3.21213203435596,2.01213203435596,2.1425)) ;
#14429=CARTESIAN_POINT('Origin',(-3.21213203435596,2.01213203435596,2.1425)) ;
#14430=CARTESIAN_POINT('Origin',(-3.,2.1,2.125)) ;
#14431=CARTESIAN_POINT('',(-3.00205541252578,2.1,2.10008463768377)) ;
#14432=CARTESIAN_POINT('',(-3.00972677312074,2.12258659483917,2.12050159825838)) ;
#14433=CARTESIAN_POINT('Origin',(-3.,2.1,2.125)) ;
#14434=CARTESIAN_POINT('',(-2.99794458747422,2.1,2.14991536231623)) ;
#14435=CARTESIAN_POINT('Origin',(-3.,2.1,2.125)) ;
#14436=CARTESIAN_POINT('Origin',(-3.,2.1,2.125)) ;
#14437=CARTESIAN_POINT('Origin',(-2.78786796564404,2.01213203435596,2.1075)) ;
#14438=CARTESIAN_POINT('',(-2.78932136177915,2.01358543049108,2.08258463768377)) ;
#14439=CARTESIAN_POINT('',(-2.78641456950892,2.01067863822085,2.13241536231623)) ;
#14440=CARTESIAN_POINT('Origin',(-2.78786796564404,2.01213203435596,2.1075)) ;
#14441=CARTESIAN_POINT('Origin',(-2.78786796564404,2.01213203435596,2.1075)) ;
#14442=CARTESIAN_POINT('Origin',(-2.7,1.8,2.09)) ;
#14443=CARTESIAN_POINT('',(-2.7,1.80205541252578,2.06508463768377)) ;
#14444=CARTESIAN_POINT('',(-2.7,1.79794458747422,2.11491536231623)) ;
#14445=CARTESIAN_POINT('Origin',(-2.7,1.8,2.09)) ;
#14446=CARTESIAN_POINT('Origin',(-2.7,1.8,2.09)) ;
#14447=CARTESIAN_POINT('Origin',(-2.78786796564404,1.58786796564404,2.0725)) ;
#14448=CARTESIAN_POINT('',(-2.78641456950892,1.58932136177915,2.04758463768377)) ;
#14449=CARTESIAN_POINT('',(-2.78932136177915,1.58641456950892,2.09741536231623)) ;
#14450=CARTESIAN_POINT('Origin',(-2.78786796564404,1.58786796564404,2.0725)) ;
#14451=CARTESIAN_POINT('Origin',(-2.78786796564404,1.58786796564404,2.0725)) ;
#14452=CARTESIAN_POINT('Origin',(-3.,1.5,2.055)) ;
#14453=CARTESIAN_POINT('',(-2.99794458747422,1.5,2.03008463768377)) ;
#14454=CARTESIAN_POINT('',(-3.00205541252578,1.5,2.07991536231623)) ;
#14455=CARTESIAN_POINT('Origin',(-3.,1.5,2.055)) ;
#14456=CARTESIAN_POINT('',(-3.00972677312074,1.47741340516083,2.05949840174162)) ;
#14457=CARTESIAN_POINT('Origin',(-3.,1.5,2.055)) ;
#14458=CARTESIAN_POINT('Origin',(-3.,1.5,2.055)) ;
#14459=CARTESIAN_POINT('Origin',(-3.21213203435596,1.58786796564404,2.0375)) ;
#14460=CARTESIAN_POINT('',(-3.21067863822085,1.58641456950892,2.01258463768377)) ;
#14461=CARTESIAN_POINT('',(-3.22185880747671,1.56528137080487,2.04199840174162)) ;
#14462=CARTESIAN_POINT('Origin',(-3.21213203435596,1.58786796564404,2.0375)) ;
#14463=CARTESIAN_POINT('',(-3.21358543049108,1.58932136177915,2.06241536231623)) ;
#14464=CARTESIAN_POINT('Origin',(-3.21213203435596,1.58786796564404,2.0375)) ;
#14465=CARTESIAN_POINT('',(-3.23524046317499,1.5783608422783,2.03828429766351)) ;
#14466=CARTESIAN_POINT('Origin',(-3.21213203435596,1.58786796564404,2.0375)) ;
#14467=CARTESIAN_POINT('Origin',(-3.21213203435596,1.58786796564404,2.0375)) ;
#14468=CARTESIAN_POINT('Origin',(-3.3,1.8,2.02)) ;
#14469=CARTESIAN_POINT('',(-3.3,1.79794458747422,1.99508463768377)) ;
#14470=CARTESIAN_POINT('',(-3.32310842881902,1.79049287663427,2.02078429766351)) ;
#14471=CARTESIAN_POINT('Origin',(-3.3,1.8,2.02)) ;
#14472=CARTESIAN_POINT('',(-3.3,1.80205541252578,2.04491536231623)) ;
#14473=CARTESIAN_POINT('Origin',(-3.3,1.8,2.02)) ;
#14474=CARTESIAN_POINT('',(-3.32310842881902,1.80950712336573,2.01921570233649)) ;
#14475=CARTESIAN_POINT('Origin',(-3.3,1.8,2.02)) ;
#14476=CARTESIAN_POINT('Origin',(-3.3,1.8,2.02)) ;
#14477=CARTESIAN_POINT('Origin',(-3.21213203435596,2.01213203435596,2.0025)) ;
#14478=CARTESIAN_POINT('',(-3.21358543049108,2.01067863822085,1.97758463768377)) ;
#14479=CARTESIAN_POINT('',(-3.23524046317499,2.0216391577217,2.00171570233649)) ;
#14480=CARTESIAN_POINT('Origin',(-3.21213203435596,2.01213203435596,2.0025)) ;
#14481=CARTESIAN_POINT('',(-3.21067863822085,2.01358543049108,2.02741536231623)) ;
#14482=CARTESIAN_POINT('Origin',(-3.21213203435596,2.01213203435596,2.0025)) ;
#14483=CARTESIAN_POINT('',(-3.22185880747671,2.03471862919513,1.99800159825838)) ;
#14484=CARTESIAN_POINT('Origin',(-3.21213203435596,2.01213203435596,2.0025)) ;
#14485=CARTESIAN_POINT('Origin',(-3.21213203435596,2.01213203435596,2.0025)) ;
#14486=CARTESIAN_POINT('Origin',(-3.,2.1,1.985)) ;
#14487=CARTESIAN_POINT('',(-3.00205541252578,2.1,1.96008463768377)) ;
#14488=CARTESIAN_POINT('',(-3.00972677312074,2.12258659483917,1.98050159825838)) ;
#14489=CARTESIAN_POINT('Origin',(-3.,2.1,1.985)) ;
#14490=CARTESIAN_POINT('',(-2.99794458747422,2.1,2.00991536231623)) ;
#14491=CARTESIAN_POINT('Origin',(-3.,2.1,1.985)) ;
#14492=CARTESIAN_POINT('Origin',(-3.,2.1,1.985)) ;
#14493=CARTESIAN_POINT('Origin',(-2.78786796564404,2.01213203435596,1.9675)) ;
#14494=CARTESIAN_POINT('',(-2.78932136177915,2.01358543049108,1.94258463768377)) ;
#14495=CARTESIAN_POINT('',(-2.78641456950892,2.01067863822085,1.99241536231623)) ;
#14496=CARTESIAN_POINT('Origin',(-2.78786796564404,2.01213203435596,1.9675)) ;
#14497=CARTESIAN_POINT('Origin',(-2.78786796564404,2.01213203435596,1.9675)) ;
#14498=CARTESIAN_POINT('Origin',(-2.74393398282202,1.69393398282202,2.36125)) ;
#14499=CARTESIAN_POINT('',(-2.72310842881902,1.80950712336573,2.37078429766351)) ;
#14500=CARTESIAN_POINT('Origin',(-2.7,1.8,2.37)) ;
#14501=CARTESIAN_POINT('',(-2.80704621154481,1.60686338991361,2.35406704255313)) ;
#14502=CARTESIAN_POINT('',(-2.76704241164104,1.70344110618775,2.36203429766351)) ;
#14503=CARTESIAN_POINT('',(-2.80699513023089,1.60656079084632,2.35622290901061)) ;
#14504=CARTESIAN_POINT('Origin',(-2.78786796564404,1.58786796564404,2.3525)) ;
#14505=CARTESIAN_POINT('Origin',(-2.78786796564404,1.58786796564404,2.3525)) ;
#14506=CARTESIAN_POINT('Origin',(-2.78786796564404,1.58786796564404,2.3525)) ;
#14507=CARTESIAN_POINT('Origin',(-2.7,1.8,2.37)) ;
#14508=CARTESIAN_POINT('Origin',(-2.89393398282202,1.54393398282202,2.34375)) ;
#14509=CARTESIAN_POINT('',(-3.00043433938457,1.52643564692014,2.34026498841428)) ;
#14510=CARTESIAN_POINT('',(-2.90366075594276,1.56652057766118,2.34824840174162)) ;
#14511=CARTESIAN_POINT('Origin',(-3.,1.5,2.335)) ;
#14512=CARTESIAN_POINT('Origin',(-3.,1.5,2.335)) ;
#14513=CARTESIAN_POINT('Origin',(-3.10606601717798,1.54393398282202,2.32625)) ;
#14514=CARTESIAN_POINT('',(-3.11579279029872,1.52134738798285,2.33074840174162)) ;
#14515=CARTESIAN_POINT('Origin',(-3.21213203435596,1.58786796564404,2.3175)) ;
#14516=CARTESIAN_POINT('Origin',(-3.25606601717798,1.69393398282202,2.30875)) ;
#14517=CARTESIAN_POINT('',(-3.279174445997,1.68442685945629,2.30953429766351)) ;
#14518=CARTESIAN_POINT('Origin',(-3.3,1.8,2.3)) ;
#14519=CARTESIAN_POINT('Origin',(-3.25606601717798,1.90606601717798,2.29125)) ;
#14520=CARTESIAN_POINT('',(-3.279174445997,1.91557314054372,2.29046570233649)) ;
#14521=CARTESIAN_POINT('Origin',(-3.21213203435596,2.01213203435596,2.2825)) ;
#14522=CARTESIAN_POINT('Origin',(-3.10606601717798,2.05606601717798,2.27375)) ;
#14523=CARTESIAN_POINT('',(-3.11579279029872,2.07865261201715,2.26925159825838)) ;
#14524=CARTESIAN_POINT('',(-3.00043433938457,2.07356435307986,2.25973501158572)) ;
#14525=CARTESIAN_POINT('Origin',(-3.,2.1,2.265)) ;
#14526=CARTESIAN_POINT('Origin',(-3.,2.1,2.265)) ;
#14527=CARTESIAN_POINT('Origin',(-2.89393398282202,2.05606601717798,2.25625)) ;
#14528=CARTESIAN_POINT('',(-2.80699513023089,1.99343920915368,2.24377709098939)) ;
#14529=CARTESIAN_POINT('',(-2.90366075594276,2.03347942233882,2.25175159825838)) ;
#14530=CARTESIAN_POINT('',(-2.80704621154481,1.99313661008639,2.24593295744687)) ;
#14531=CARTESIAN_POINT('Origin',(-2.78786796564404,2.01213203435596,2.2475)) ;
#14532=CARTESIAN_POINT('Origin',(-2.78786796564404,2.01213203435596,2.2475)) ;
#14533=CARTESIAN_POINT('Origin',(-2.78786796564404,2.01213203435596,2.2475)) ;
#14534=CARTESIAN_POINT('Origin',(-2.74393398282202,1.90606601717798,2.23875)) ;
#14535=CARTESIAN_POINT('',(-2.72704640825626,1.8,2.23)) ;
#14536=CARTESIAN_POINT('',(-2.76704241164104,1.89655889381225,2.23796570233649)) ;
#14537=CARTESIAN_POINT('Origin',(-2.7,1.8,2.23)) ;
#14538=CARTESIAN_POINT('Origin',(-2.7,1.8,2.23)) ;
#14539=CARTESIAN_POINT('Origin',(-2.74393398282202,1.69393398282202,2.22125)) ;
#14540=CARTESIAN_POINT('',(-2.80704621154481,1.60686338991361,2.21406704255313)) ;
#14541=CARTESIAN_POINT('',(-2.76704241164104,1.70344110618775,2.22203429766351)) ;
#14542=CARTESIAN_POINT('',(-2.80699513023089,1.60656079084632,2.21622290901061)) ;
#14543=CARTESIAN_POINT('Origin',(-2.78786796564404,1.58786796564404,2.2125)) ;
#14544=CARTESIAN_POINT('Origin',(-2.78786796564404,1.58786796564404,2.2125)) ;
#14545=CARTESIAN_POINT('Origin',(-2.78786796564404,1.58786796564404,2.2125)) ;
#14546=CARTESIAN_POINT('Origin',(-2.89393398282202,1.54393398282202,2.20375)) ;
#14547=CARTESIAN_POINT('',(-3.00043433938457,1.52643564692014,2.20026498841428)) ;
#14548=CARTESIAN_POINT('',(-2.90366075594276,1.56652057766118,2.20824840174162)) ;
#14549=CARTESIAN_POINT('Origin',(-3.,1.5,2.195)) ;
#14550=CARTESIAN_POINT('Origin',(-3.,1.5,2.195)) ;
#14551=CARTESIAN_POINT('Origin',(-3.10606601717798,1.54393398282202,2.18625)) ;
#14552=CARTESIAN_POINT('',(-3.11579279029872,1.52134738798285,2.19074840174162)) ;
#14553=CARTESIAN_POINT('Origin',(-3.21213203435596,1.58786796564404,2.1775)) ;
#14554=CARTESIAN_POINT('Origin',(-3.25606601717798,1.69393398282202,2.16875)) ;
#14555=CARTESIAN_POINT('',(-3.279174445997,1.68442685945629,2.16953429766351)) ;
#14556=CARTESIAN_POINT('Origin',(-3.3,1.8,2.16)) ;
#14557=CARTESIAN_POINT('Origin',(-3.25606601717798,1.90606601717798,2.15125)) ;
#14558=CARTESIAN_POINT('',(-3.279174445997,1.91557314054372,2.15046570233649)) ;
#14559=CARTESIAN_POINT('Origin',(-3.21213203435596,2.01213203435596,2.1425)) ;
#14560=CARTESIAN_POINT('Origin',(-3.10606601717798,2.05606601717798,2.13375)) ;
#14561=CARTESIAN_POINT('',(-3.11579279029872,2.07865261201715,2.12925159825838)) ;
#14562=CARTESIAN_POINT('',(-3.00043433938457,2.07356435307986,2.11973501158572)) ;
#14563=CARTESIAN_POINT('Origin',(-3.,2.1,2.125)) ;
#14564=CARTESIAN_POINT('Origin',(-3.,2.1,2.125)) ;
#14565=CARTESIAN_POINT('Origin',(-2.89393398282202,2.05606601717798,2.11625)) ;
#14566=CARTESIAN_POINT('',(-2.80699513023089,1.99343920915368,2.10377709098939)) ;
#14567=CARTESIAN_POINT('',(-2.90366075594276,2.03347942233882,2.11175159825838)) ;
#14568=CARTESIAN_POINT('',(-2.80704621154481,1.99313661008639,2.10593295744687)) ;
#14569=CARTESIAN_POINT('Origin',(-2.78786796564404,2.01213203435596,2.1075)) ;
#14570=CARTESIAN_POINT('Origin',(-2.78786796564404,2.01213203435596,2.1075)) ;
#14571=CARTESIAN_POINT('Origin',(-2.78786796564404,2.01213203435596,2.1075)) ;
#14572=CARTESIAN_POINT('Origin',(-2.74393398282202,1.90606601717798,2.09875)) ;
#14573=CARTESIAN_POINT('',(-2.72704640825626,1.8,2.09)) ;
#14574=CARTESIAN_POINT('',(-2.76704241164104,1.89655889381225,2.09796570233649)) ;
#14575=CARTESIAN_POINT('Origin',(-2.7,1.8,2.09)) ;
#14576=CARTESIAN_POINT('Origin',(-2.7,1.8,2.09)) ;
#14577=CARTESIAN_POINT('Origin',(-2.74393398282202,1.69393398282202,2.08125)) ;
#14578=CARTESIAN_POINT('',(-2.80704621154481,1.60686338991361,2.07406704255313)) ;
#14579=CARTESIAN_POINT('',(-2.76704241164104,1.70344110618775,2.08203429766351)) ;
#14580=CARTESIAN_POINT('',(-2.80699513023089,1.60656079084632,2.07622290901061)) ;
#14581=CARTESIAN_POINT('Origin',(-2.78786796564404,1.58786796564404,2.0725)) ;
#14582=CARTESIAN_POINT('Origin',(-2.78786796564404,1.58786796564404,2.0725)) ;
#14583=CARTESIAN_POINT('Origin',(-2.78786796564404,1.58786796564404,2.0725)) ;
#14584=CARTESIAN_POINT('Origin',(-2.89393398282202,1.54393398282202,2.06375)) ;
#14585=CARTESIAN_POINT('',(-3.00043433938457,1.52643564692014,2.06026498841428)) ;
#14586=CARTESIAN_POINT('',(-2.90366075594276,1.56652057766118,2.06824840174162)) ;
#14587=CARTESIAN_POINT('Origin',(-3.,1.5,2.055)) ;
#14588=CARTESIAN_POINT('Origin',(-3.,1.5,2.055)) ;
#14589=CARTESIAN_POINT('Origin',(-3.10606601717798,1.54393398282202,2.04625)) ;
#14590=CARTESIAN_POINT('',(-3.11579279029872,1.52134738798285,2.05074840174162)) ;
#14591=CARTESIAN_POINT('Origin',(-3.21213203435596,1.58786796564404,2.0375)) ;
#14592=CARTESIAN_POINT('Origin',(-3.25606601717798,1.69393398282202,2.02875)) ;
#14593=CARTESIAN_POINT('',(-3.279174445997,1.68442685945629,2.02953429766351)) ;
#14594=CARTESIAN_POINT('Origin',(-3.3,1.8,2.02)) ;
#14595=CARTESIAN_POINT('Origin',(-3.25606601717798,1.90606601717798,2.01125)) ;
#14596=CARTESIAN_POINT('',(-3.279174445997,1.91557314054371,2.01046570233649)) ;
#14597=CARTESIAN_POINT('Origin',(-3.21213203435596,2.01213203435596,2.0025)) ;
#14598=CARTESIAN_POINT('Origin',(-3.10606601717798,2.05606601717798,1.99375)) ;
#14599=CARTESIAN_POINT('',(-3.11579279029872,2.07865261201715,1.98925159825838)) ;
#14600=CARTESIAN_POINT('',(-3.00043433938457,2.07356435307986,1.97973501158572)) ;
#14601=CARTESIAN_POINT('Origin',(-3.,2.1,1.985)) ;
#14602=CARTESIAN_POINT('Origin',(-3.,2.1,1.985)) ;
#14603=CARTESIAN_POINT('Origin',(-2.89393398282202,2.05606601717798,1.97625)) ;
#14604=CARTESIAN_POINT('',(-2.80699513023089,1.99343920915368,1.96377709098939)) ;
#14605=CARTESIAN_POINT('',(-2.90366075594276,2.03347942233882,1.97175159825838)) ;
#14606=CARTESIAN_POINT('',(-2.80704621154481,1.99313661008639,1.96593295744687)) ;
#14607=CARTESIAN_POINT('Origin',(-2.78786796564404,2.01213203435596,1.9675)) ;
#14608=CARTESIAN_POINT('Origin',(-2.78786796564404,2.01213203435596,1.9675)) ;
#14609=CARTESIAN_POINT('Origin',(-2.78786796564404,2.01213203435596,1.9675)) ;
#14610=CARTESIAN_POINT('Origin',(-2.74393398282202,1.90606601717798,1.95875)) ;
#14611=CARTESIAN_POINT('',(-2.72310842881902,1.79049287663427,1.94921570233649)) ;
#14612=CARTESIAN_POINT('',(-2.76704241164104,1.89655889381225,1.95796570233649)) ;
#14613=CARTESIAN_POINT('Origin',(-2.7,1.8,1.95)) ;
#14614=CARTESIAN_POINT('Origin',(-2.7,1.8,1.95)) ;
#15424=UNCERTAINTY_MEASURE_WITH_UNIT(LENGTH_MEASURE(0.001),#15485,
'DISTANCE_ACCURACY_VALUE',
'Maximum model space distance between geometric entities at asserted c
onnectivities') ;
#15441=UNCERTAINTY_MEASURE_WITH_UNIT(LENGTH_MEASURE(0.001),#15485,
'DISTANCE_ACCURACY_VALUE',
'Maximum model space distance between geometric entities at asserted c
onnectivities') ;
#15467=(
GEOMETRIC_REPRESENTATION_CONTEXT(3)
GLOBAL_UNCERTAINTY_ASSIGNED_CONTEXT((#15424))
GLOBAL_UNIT_ASSIGNED_CONTEXT((#15485,#15487,#15488))
REPRESENTATION_CONTEXT('','3D')
) ;
#15484=(
GEOMETRIC_REPRESENTATION_CONTEXT(3)
GLOBAL_UNCERTAINTY_ASSIGNED_CONTEXT((#15441))
GLOBAL_UNIT_ASSIGNED_CONTEXT((#15485,#15487,#15488))
REPRESENTATION_CONTEXT('','3D')
) ;
#15485=(
LENGTH_UNIT()
NAMED_UNIT(*)
SI_UNIT(.CENTI.,.METRE.)
) ;
#15487=(
NAMED_UNIT(*)
PLANE_ANGLE_UNIT()
SI_UNIT($,.RADIAN.)
) ;
#15488=(
NAMED_UNIT(*)
SI_UNIT($,.STERADIAN.)
SOLID_ANGLE_UNIT()
) ;
#15514=SHAPE_DEFINITION_REPRESENTATION(#15571,#15643) ;
#15571=PRODUCT_DEFINITION_SHAPE('',$,#15686) ;
#15643=SHAPE_REPRESENTATION('',(#9349),#15467) ;
#15660=PRODUCT_DEFINITION_CONTEXT('part definition',#15788,'design') ;
#15686=PRODUCT_DEFINITION('BUTTON_RETURN_SPRING',
'BUTTON_RETURN_SPRING',#15728,#15660) ;
#15728=PRODUCT_DEFINITION_FORMATION('',$,#15815) ;
#15788=APPLICATION_CONTEXT(
'Core Data for Automotive Mechanical Design Process') ;
#15789=PRODUCT_CONTEXT('part definition',#15788,'mechanical') ;
#15815=PRODUCT('BUTTON_RETURN_SPRING','BUTTON_RETURN_SPRING',$,(#15789)) ;
#15832=PRESENTATION_STYLE_ASSIGNMENT((#15844)) ;
#15844=SURFACE_STYLE_USAGE(.BOTH.,#15856) ;
#15856=SURFACE_SIDE_STYLE('',(#15868)) ;
#15868=SURFACE_STYLE_FILL_AREA(#15880) ;
#15880=FILL_AREA_STYLE('Steel - Satin',(#15892)) ;
#15892=FILL_AREA_STYLE_COLOUR('Steel - Satin',#15904) ;
#15904=COLOUR_RGB('Steel - Satin', 0.72549020, 0.75294118, 0.79215686) ;
ENDSEC;
END-ISO-10303-21;
